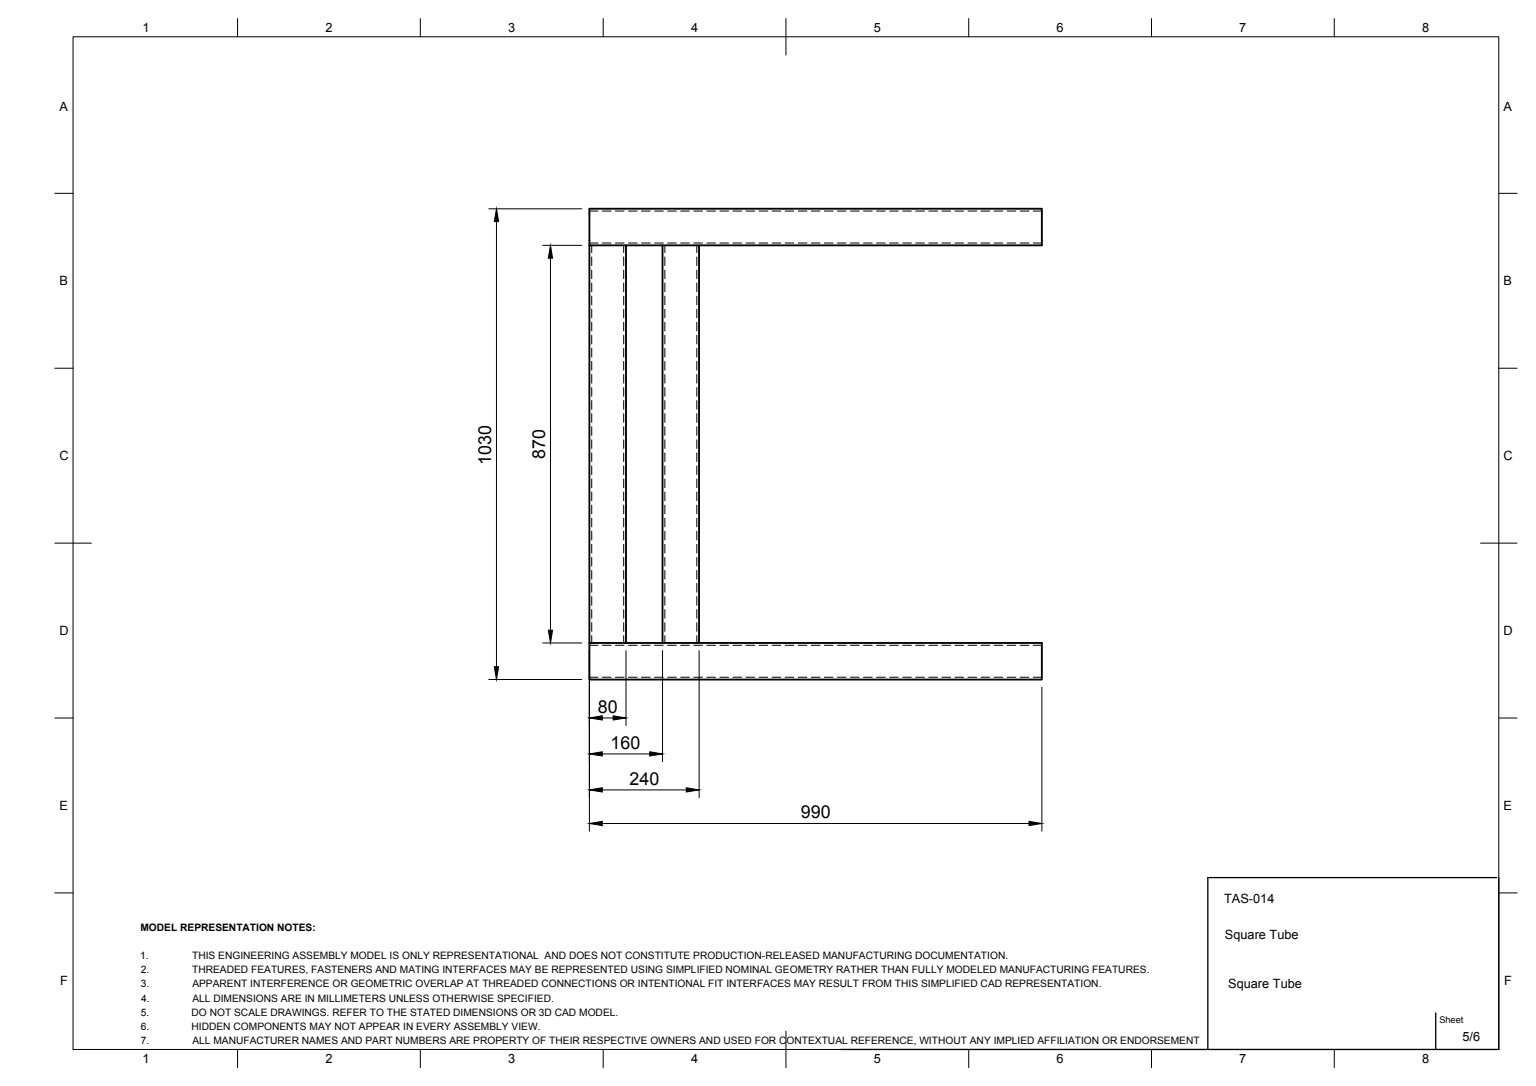
ISO-10303-21;
HEADER;
/* Generated by software containing ST-Developer
 * from STEP Tools, Inc. (www.steptools.com) 
 */

FILE_DESCRIPTION(
/* description */ ('STEP AP214'),
/* implementation_level */ '2;1');

FILE_NAME(
/* name */ 'Square Tube.step',
/* time_stamp */ '2026-11-15T15:22:30-08:00',
/* author */ (''),
/* organization */ (''),
/* preprocessor_version */ 'ST-DEVELOPER v20.2',
/* originating_system */ 'Autodesk Translation Framework v15.17.0.0',
/* authorisation */ '');

FILE_SCHEMA (('AUTOMOTIVE_DESIGN { 1 0 10303 214 3 1 1 }'));
ENDSEC;

DATA;
#10=MECHANICAL_DESIGN_GEOMETRIC_PRESENTATION_REPRESENTATION('',(#79,#80,#81,#82,#83,#84),#3119);
#67=SHAPE_REPRESENTATION_RELATIONSHIP('SRR','None',#3149,#71);
#71=ADVANCED_BREP_SHAPE_REPRESENTATION('',(#88,#89,#90,#91),#3115);
#75=OPEN_SHELL('',(#1779));
#76=OPEN_SHELL('',(#1780));
#77=SHELL_BASED_SURFACE_MODEL('Body5',(#75));
#78=SHELL_BASED_SURFACE_MODEL('Body6',(#76));
#79=STYLED_ITEM('',(#3178),#88);
#80=STYLED_ITEM('',(#3178),#89);
#81=STYLED_ITEM('',(#3178),#90);
#82=STYLED_ITEM('',(#3178),#91);
#83=STYLED_ITEM('',(#3178),#77);
#84=STYLED_ITEM('',(#3178),#78);
#88=MANIFOLD_SOLID_BREP('Body1',#1800);
#89=MANIFOLD_SOLID_BREP('Body2',#1801);
#90=MANIFOLD_SOLID_BREP('Body3',#1802);
#91=MANIFOLD_SOLID_BREP('Body4',#1803);
#95=FACE_BOUND('',#317,.T.);
#96=FACE_BOUND('',#319,.T.);
#97=FACE_BOUND('',#337,.T.);
#98=FACE_BOUND('',#339,.T.);
#99=FACE_BOUND('',#357,.T.);
#100=FACE_BOUND('',#359,.T.);
#101=FACE_BOUND('',#377,.T.);
#102=FACE_BOUND('',#379,.T.);
#103=CIRCLE('',#1856,5.);
#104=CIRCLE('',#1857,5.);
#105=CIRCLE('',#1860,5.);
#106=CIRCLE('',#1861,5.);
#107=CIRCLE('',#1864,5.);
#108=CIRCLE('',#1865,5.);
#109=CIRCLE('',#1868,5.);
#110=CIRCLE('',#1869,5.);
#111=CIRCLE('',#1872,10.);
#112=CIRCLE('',#1873,10.);
#113=CIRCLE('',#1876,10.);
#114=CIRCLE('',#1877,10.);
#115=CIRCLE('',#1880,10.);
#116=CIRCLE('',#1881,10.);
#117=CIRCLE('',#1884,10.);
#118=CIRCLE('',#1885,10.);
#119=CIRCLE('',#1890,5.);
#120=CIRCLE('',#1891,5.);
#121=CIRCLE('',#1894,5.);
#122=CIRCLE('',#1895,5.);
#123=CIRCLE('',#1898,5.);
#124=CIRCLE('',#1899,5.);
#125=CIRCLE('',#1902,5.);
#126=CIRCLE('',#1903,5.);
#127=CIRCLE('',#1906,10.);
#128=CIRCLE('',#1907,10.);
#129=CIRCLE('',#1910,10.);
#130=CIRCLE('',#1911,10.);
#131=CIRCLE('',#1914,10.);
#132=CIRCLE('',#1915,10.);
#133=CIRCLE('',#1918,10.);
#134=CIRCLE('',#1919,10.);
#135=CIRCLE('',#1923,10.);
#136=CIRCLE('',#1924,10.);
#137=CIRCLE('',#1927,10.);
#138=CIRCLE('',#1928,10.);
#139=CIRCLE('',#1931,10.);
#140=CIRCLE('',#1932,10.);
#141=CIRCLE('',#1935,10.);
#142=CIRCLE('',#1936,10.);
#143=CIRCLE('',#1938,5.);
#144=CIRCLE('',#1939,5.);
#145=CIRCLE('',#1942,5.);
#146=CIRCLE('',#1943,5.);
#147=CIRCLE('',#1946,5.);
#148=CIRCLE('',#1947,5.);
#149=CIRCLE('',#1950,5.);
#150=CIRCLE('',#1951,5.);
#151=CIRCLE('',#1957,10.);
#152=CIRCLE('',#1958,10.);
#153=CIRCLE('',#1961,10.);
#154=CIRCLE('',#1962,10.);
#155=CIRCLE('',#1965,10.);
#156=CIRCLE('',#1966,10.);
#157=CIRCLE('',#1969,10.);
#158=CIRCLE('',#1970,10.);
#159=CIRCLE('',#1972,5.);
#160=CIRCLE('',#1973,5.);
#161=CIRCLE('',#1976,5.);
#162=CIRCLE('',#1977,5.);
#163=CIRCLE('',#1980,5.);
#164=CIRCLE('',#1981,5.);
#165=CIRCLE('',#1984,5.);
#166=CIRCLE('',#1985,5.);
#167=CIRCLE('',#1991,5.);
#168=CIRCLE('',#1992,5.);
#169=CIRCLE('',#1993,5.);
#170=CIRCLE('',#1994,5.);
#171=CIRCLE('',#1996,5.);
#172=CIRCLE('',#1997,5.);
#173=CIRCLE('',#1998,5.);
#174=CIRCLE('',#1999,5.);
#175=CYLINDRICAL_SURFACE('',#1855,5.);
#176=CYLINDRICAL_SURFACE('',#1859,5.);
#177=CYLINDRICAL_SURFACE('',#1863,5.);
#178=CYLINDRICAL_SURFACE('',#1867,5.);
#179=CYLINDRICAL_SURFACE('',#1871,10.);
#180=CYLINDRICAL_SURFACE('',#1875,10.);
#181=CYLINDRICAL_SURFACE('',#1879,10.);
#182=CYLINDRICAL_SURFACE('',#1883,10.);
#183=CYLINDRICAL_SURFACE('',#1889,5.);
#184=CYLINDRICAL_SURFACE('',#1893,5.);
#185=CYLINDRICAL_SURFACE('',#1897,5.);
#186=CYLINDRICAL_SURFACE('',#1901,5.);
#187=CYLINDRICAL_SURFACE('',#1905,10.);
#188=CYLINDRICAL_SURFACE('',#1909,10.);
#189=CYLINDRICAL_SURFACE('',#1913,10.);
#190=CYLINDRICAL_SURFACE('',#1917,10.);
#191=CYLINDRICAL_SURFACE('',#1922,10.);
#192=CYLINDRICAL_SURFACE('',#1926,10.);
#193=CYLINDRICAL_SURFACE('',#1930,10.);
#194=CYLINDRICAL_SURFACE('',#1934,10.);
#195=CYLINDRICAL_SURFACE('',#1937,5.);
#196=CYLINDRICAL_SURFACE('',#1941,5.);
#197=CYLINDRICAL_SURFACE('',#1945,5.);
#198=CYLINDRICAL_SURFACE('',#1949,5.);
#199=CYLINDRICAL_SURFACE('',#1956,10.);
#200=CYLINDRICAL_SURFACE('',#1960,10.);
#201=CYLINDRICAL_SURFACE('',#1964,10.);
#202=CYLINDRICAL_SURFACE('',#1968,10.);
#203=CYLINDRICAL_SURFACE('',#1971,5.);
#204=CYLINDRICAL_SURFACE('',#1975,5.);
#205=CYLINDRICAL_SURFACE('',#1979,5.);
#206=CYLINDRICAL_SURFACE('',#1983,5.);
#207=FACE_OUTER_BOUND('',#300,.T.);
#208=FACE_OUTER_BOUND('',#301,.T.);
#209=FACE_OUTER_BOUND('',#302,.T.);
#210=FACE_OUTER_BOUND('',#303,.T.);
#211=FACE_OUTER_BOUND('',#304,.T.);
#212=FACE_OUTER_BOUND('',#305,.T.);
#213=FACE_OUTER_BOUND('',#306,.T.);
#214=FACE_OUTER_BOUND('',#307,.T.);
#215=FACE_OUTER_BOUND('',#308,.T.);
#216=FACE_OUTER_BOUND('',#309,.T.);
#217=FACE_OUTER_BOUND('',#310,.T.);
#218=FACE_OUTER_BOUND('',#311,.T.);
#219=FACE_OUTER_BOUND('',#312,.T.);
#220=FACE_OUTER_BOUND('',#313,.T.);
#221=FACE_OUTER_BOUND('',#314,.T.);
#222=FACE_OUTER_BOUND('',#315,.T.);
#223=FACE_OUTER_BOUND('',#316,.T.);
#224=FACE_OUTER_BOUND('',#318,.T.);
#225=FACE_OUTER_BOUND('',#320,.T.);
#226=FACE_OUTER_BOUND('',#321,.T.);
#227=FACE_OUTER_BOUND('',#322,.T.);
#228=FACE_OUTER_BOUND('',#323,.T.);
#229=FACE_OUTER_BOUND('',#324,.T.);
#230=FACE_OUTER_BOUND('',#325,.T.);
#231=FACE_OUTER_BOUND('',#326,.T.);
#232=FACE_OUTER_BOUND('',#327,.T.);
#233=FACE_OUTER_BOUND('',#328,.T.);
#234=FACE_OUTER_BOUND('',#329,.T.);
#235=FACE_OUTER_BOUND('',#330,.T.);
#236=FACE_OUTER_BOUND('',#331,.T.);
#237=FACE_OUTER_BOUND('',#332,.T.);
#238=FACE_OUTER_BOUND('',#333,.T.);
#239=FACE_OUTER_BOUND('',#334,.T.);
#240=FACE_OUTER_BOUND('',#335,.T.);
#241=FACE_OUTER_BOUND('',#336,.T.);
#242=FACE_OUTER_BOUND('',#338,.T.);
#243=FACE_OUTER_BOUND('',#340,.T.);
#244=FACE_OUTER_BOUND('',#341,.T.);
#245=FACE_OUTER_BOUND('',#342,.T.);
#246=FACE_OUTER_BOUND('',#343,.T.);
#247=FACE_OUTER_BOUND('',#344,.T.);
#248=FACE_OUTER_BOUND('',#345,.T.);
#249=FACE_OUTER_BOUND('',#346,.T.);
#250=FACE_OUTER_BOUND('',#347,.T.);
#251=FACE_OUTER_BOUND('',#348,.T.);
#252=FACE_OUTER_BOUND('',#349,.T.);
#253=FACE_OUTER_BOUND('',#350,.T.);
#254=FACE_OUTER_BOUND('',#351,.T.);
#255=FACE_OUTER_BOUND('',#352,.T.);
#256=FACE_OUTER_BOUND('',#353,.T.);
#257=FACE_OUTER_BOUND('',#354,.T.);
#258=FACE_OUTER_BOUND('',#355,.T.);
#259=FACE_OUTER_BOUND('',#356,.T.);
#260=FACE_OUTER_BOUND('',#358,.T.);
#261=FACE_OUTER_BOUND('',#360,.T.);
#262=FACE_OUTER_BOUND('',#361,.T.);
#263=FACE_OUTER_BOUND('',#362,.T.);
#264=FACE_OUTER_BOUND('',#363,.T.);
#265=FACE_OUTER_BOUND('',#364,.T.);
#266=FACE_OUTER_BOUND('',#365,.T.);
#267=FACE_OUTER_BOUND('',#366,.T.);
#268=FACE_OUTER_BOUND('',#367,.T.);
#269=FACE_OUTER_BOUND('',#368,.T.);
#270=FACE_OUTER_BOUND('',#369,.T.);
#271=FACE_OUTER_BOUND('',#370,.T.);
#272=FACE_OUTER_BOUND('',#371,.T.);
#273=FACE_OUTER_BOUND('',#372,.T.);
#274=FACE_OUTER_BOUND('',#373,.T.);
#275=FACE_OUTER_BOUND('',#374,.T.);
#276=FACE_OUTER_BOUND('',#375,.T.);
#277=FACE_OUTER_BOUND('',#376,.T.);
#278=FACE_OUTER_BOUND('',#378,.T.);
#279=FACE_OUTER_BOUND('',#380,.T.);
#280=FACE_OUTER_BOUND('',#381,.T.);
#300=EDGE_LOOP('',(#1168,#1169,#1170,#1171));
#301=EDGE_LOOP('',(#1172,#1173,#1174,#1175));
#302=EDGE_LOOP('',(#1176,#1177,#1178,#1179));
#303=EDGE_LOOP('',(#1180,#1181,#1182,#1183));
#304=EDGE_LOOP('',(#1184,#1185,#1186,#1187));
#305=EDGE_LOOP('',(#1188,#1189,#1190,#1191));
#306=EDGE_LOOP('',(#1192,#1193,#1194,#1195));
#307=EDGE_LOOP('',(#1196,#1197,#1198,#1199));
#308=EDGE_LOOP('',(#1200,#1201,#1202,#1203));
#309=EDGE_LOOP('',(#1204,#1205,#1206,#1207));
#310=EDGE_LOOP('',(#1208,#1209,#1210,#1211));
#311=EDGE_LOOP('',(#1212,#1213,#1214,#1215));
#312=EDGE_LOOP('',(#1216,#1217,#1218,#1219));
#313=EDGE_LOOP('',(#1220,#1221,#1222,#1223));
#314=EDGE_LOOP('',(#1224,#1225,#1226,#1227));
#315=EDGE_LOOP('',(#1228,#1229,#1230,#1231));
#316=EDGE_LOOP('',(#1232,#1233,#1234,#1235,#1236,#1237,#1238,#1239));
#317=EDGE_LOOP('',(#1240,#1241,#1242,#1243,#1244,#1245,#1246,#1247));
#318=EDGE_LOOP('',(#1248,#1249,#1250,#1251,#1252,#1253,#1254,#1255));
#319=EDGE_LOOP('',(#1256,#1257,#1258,#1259,#1260,#1261,#1262,#1263));
#320=EDGE_LOOP('',(#1264,#1265,#1266,#1267));
#321=EDGE_LOOP('',(#1268,#1269,#1270,#1271));
#322=EDGE_LOOP('',(#1272,#1273,#1274,#1275));
#323=EDGE_LOOP('',(#1276,#1277,#1278,#1279));
#324=EDGE_LOOP('',(#1280,#1281,#1282,#1283));
#325=EDGE_LOOP('',(#1284,#1285,#1286,#1287));
#326=EDGE_LOOP('',(#1288,#1289,#1290,#1291));
#327=EDGE_LOOP('',(#1292,#1293,#1294,#1295));
#328=EDGE_LOOP('',(#1296,#1297,#1298,#1299));
#329=EDGE_LOOP('',(#1300,#1301,#1302,#1303));
#330=EDGE_LOOP('',(#1304,#1305,#1306,#1307));
#331=EDGE_LOOP('',(#1308,#1309,#1310,#1311));
#332=EDGE_LOOP('',(#1312,#1313,#1314,#1315));
#333=EDGE_LOOP('',(#1316,#1317,#1318,#1319));
#334=EDGE_LOOP('',(#1320,#1321,#1322,#1323));
#335=EDGE_LOOP('',(#1324,#1325,#1326,#1327));
#336=EDGE_LOOP('',(#1328,#1329,#1330,#1331,#1332,#1333,#1334,#1335));
#337=EDGE_LOOP('',(#1336,#1337,#1338,#1339,#1340,#1341,#1342,#1343));
#338=EDGE_LOOP('',(#1344,#1345,#1346,#1347,#1348,#1349,#1350,#1351));
#339=EDGE_LOOP('',(#1352,#1353,#1354,#1355,#1356,#1357,#1358,#1359));
#340=EDGE_LOOP('',(#1360,#1361,#1362,#1363));
#341=EDGE_LOOP('',(#1364,#1365,#1366,#1367));
#342=EDGE_LOOP('',(#1368,#1369,#1370,#1371));
#343=EDGE_LOOP('',(#1372,#1373,#1374,#1375));
#344=EDGE_LOOP('',(#1376,#1377,#1378,#1379));
#345=EDGE_LOOP('',(#1380,#1381,#1382,#1383));
#346=EDGE_LOOP('',(#1384,#1385,#1386,#1387));
#347=EDGE_LOOP('',(#1388,#1389,#1390,#1391));
#348=EDGE_LOOP('',(#1392,#1393,#1394,#1395));
#349=EDGE_LOOP('',(#1396,#1397,#1398,#1399));
#350=EDGE_LOOP('',(#1400,#1401,#1402,#1403));
#351=EDGE_LOOP('',(#1404,#1405,#1406,#1407));
#352=EDGE_LOOP('',(#1408,#1409,#1410,#1411));
#353=EDGE_LOOP('',(#1412,#1413,#1414,#1415));
#354=EDGE_LOOP('',(#1416,#1417,#1418,#1419));
#355=EDGE_LOOP('',(#1420,#1421,#1422,#1423));
#356=EDGE_LOOP('',(#1424,#1425,#1426,#1427,#1428,#1429,#1430,#1431));
#357=EDGE_LOOP('',(#1432,#1433,#1434,#1435,#1436,#1437,#1438,#1439));
#358=EDGE_LOOP('',(#1440,#1441,#1442,#1443,#1444,#1445,#1446,#1447));
#359=EDGE_LOOP('',(#1448,#1449,#1450,#1451,#1452,#1453,#1454,#1455));
#360=EDGE_LOOP('',(#1456,#1457,#1458,#1459));
#361=EDGE_LOOP('',(#1460,#1461,#1462,#1463));
#362=EDGE_LOOP('',(#1464,#1465,#1466,#1467));
#363=EDGE_LOOP('',(#1468,#1469,#1470,#1471));
#364=EDGE_LOOP('',(#1472,#1473,#1474,#1475));
#365=EDGE_LOOP('',(#1476,#1477,#1478,#1479));
#366=EDGE_LOOP('',(#1480,#1481,#1482,#1483));
#367=EDGE_LOOP('',(#1484,#1485,#1486,#1487));
#368=EDGE_LOOP('',(#1488,#1489,#1490,#1491));
#369=EDGE_LOOP('',(#1492,#1493,#1494,#1495));
#370=EDGE_LOOP('',(#1496,#1497,#1498,#1499));
#371=EDGE_LOOP('',(#1500,#1501,#1502,#1503));
#372=EDGE_LOOP('',(#1504,#1505,#1506,#1507));
#373=EDGE_LOOP('',(#1508,#1509,#1510,#1511));
#374=EDGE_LOOP('',(#1512,#1513,#1514,#1515));
#375=EDGE_LOOP('',(#1516,#1517,#1518,#1519));
#376=EDGE_LOOP('',(#1520,#1521,#1522,#1523,#1524,#1525,#1526,#1527));
#377=EDGE_LOOP('',(#1528,#1529,#1530,#1531,#1532,#1533,#1534,#1535));
#378=EDGE_LOOP('',(#1536,#1537,#1538,#1539,#1540,#1541,#1542,#1543));
#379=EDGE_LOOP('',(#1544,#1545,#1546,#1547,#1548,#1549,#1550,#1551));
#380=EDGE_LOOP('',(#1552,#1553,#1554,#1555,#1556,#1557,#1558,#1559));
#381=EDGE_LOOP('',(#1560,#1561,#1562,#1563,#1564,#1565,#1566,#1567));
#401=LINE('',#2584,#576);
#402=LINE('',#2586,#577);
#403=LINE('',#2588,#578);
#404=LINE('',#2589,#579);
#405=LINE('',#2593,#580);
#406=LINE('',#2599,#581);
#407=LINE('',#2600,#582);
#408=LINE('',#2601,#583);
#409=LINE('',#2605,#584);
#410=LINE('',#2611,#585);
#411=LINE('',#2612,#586);
#412=LINE('',#2613,#587);
#413=LINE('',#2617,#588);
#414=LINE('',#2623,#589);
#415=LINE('',#2624,#590);
#416=LINE('',#2625,#591);
#417=LINE('',#2632,#592);
#418=LINE('',#2634,#593);
#419=LINE('',#2636,#594);
#420=LINE('',#2637,#595);
#421=LINE('',#2643,#596);
#422=LINE('',#2646,#597);
#423=LINE('',#2648,#598);
#424=LINE('',#2649,#599);
#425=LINE('',#2655,#600);
#426=LINE('',#2658,#601);
#427=LINE('',#2660,#602);
#428=LINE('',#2661,#603);
#429=LINE('',#2667,#604);
#430=LINE('',#2670,#605);
#431=LINE('',#2672,#606);
#432=LINE('',#2673,#607);
#433=LINE('',#2682,#608);
#434=LINE('',#2684,#609);
#435=LINE('',#2686,#610);
#436=LINE('',#2687,#611);
#437=LINE('',#2691,#612);
#438=LINE('',#2697,#613);
#439=LINE('',#2698,#614);
#440=LINE('',#2699,#615);
#441=LINE('',#2703,#616);
#442=LINE('',#2709,#617);
#443=LINE('',#2710,#618);
#444=LINE('',#2711,#619);
#445=LINE('',#2715,#620);
#446=LINE('',#2721,#621);
#447=LINE('',#2722,#622);
#448=LINE('',#2723,#623);
#449=LINE('',#2730,#624);
#450=LINE('',#2732,#625);
#451=LINE('',#2734,#626);
#452=LINE('',#2735,#627);
#453=LINE('',#2741,#628);
#454=LINE('',#2744,#629);
#455=LINE('',#2746,#630);
#456=LINE('',#2747,#631);
#457=LINE('',#2753,#632);
#458=LINE('',#2756,#633);
#459=LINE('',#2758,#634);
#460=LINE('',#2759,#635);
#461=LINE('',#2765,#636);
#462=LINE('',#2768,#637);
#463=LINE('',#2770,#638);
#464=LINE('',#2771,#639);
#465=LINE('',#2782,#640);
#466=LINE('',#2785,#641);
#467=LINE('',#2788,#642);
#468=LINE('',#2790,#643);
#469=LINE('',#2791,#644);
#470=LINE('',#2797,#645);
#471=LINE('',#2800,#646);
#472=LINE('',#2802,#647);
#473=LINE('',#2803,#648);
#474=LINE('',#2809,#649);
#475=LINE('',#2812,#650);
#476=LINE('',#2814,#651);
#477=LINE('',#2815,#652);
#478=LINE('',#2821,#653);
#479=LINE('',#2825,#654);
#480=LINE('',#2829,#655);
#481=LINE('',#2834,#656);
#482=LINE('',#2835,#657);
#483=LINE('',#2836,#658);
#484=LINE('',#2840,#659);
#485=LINE('',#2846,#660);
#486=LINE('',#2847,#661);
#487=LINE('',#2848,#662);
#488=LINE('',#2852,#663);
#489=LINE('',#2858,#664);
#490=LINE('',#2859,#665);
#491=LINE('',#2860,#666);
#492=LINE('',#2864,#667);
#493=LINE('',#2868,#668);
#494=LINE('',#2869,#669);
#495=LINE('',#2871,#670);
#496=LINE('',#2872,#671);
#497=LINE('',#2880,#672);
#498=LINE('',#2883,#673);
#499=LINE('',#2886,#674);
#500=LINE('',#2888,#675);
#501=LINE('',#2889,#676);
#502=LINE('',#2895,#677);
#503=LINE('',#2898,#678);
#504=LINE('',#2900,#679);
#505=LINE('',#2901,#680);
#506=LINE('',#2907,#681);
#507=LINE('',#2910,#682);
#508=LINE('',#2912,#683);
#509=LINE('',#2913,#684);
#510=LINE('',#2919,#685);
#511=LINE('',#2923,#686);
#512=LINE('',#2927,#687);
#513=LINE('',#2932,#688);
#514=LINE('',#2933,#689);
#515=LINE('',#2934,#690);
#516=LINE('',#2938,#691);
#517=LINE('',#2944,#692);
#518=LINE('',#2945,#693);
#519=LINE('',#2946,#694);
#520=LINE('',#2950,#695);
#521=LINE('',#2956,#696);
#522=LINE('',#2957,#697);
#523=LINE('',#2958,#698);
#524=LINE('',#2962,#699);
#525=LINE('',#2966,#700);
#526=LINE('',#2967,#701);
#527=LINE('',#2969,#702);
#528=LINE('',#2970,#703);
#529=LINE('',#2978,#704);
#530=LINE('',#2982,#705);
#531=LINE('',#2986,#706);
#532=LINE('',#2989,#707);
#533=LINE('',#2993,#708);
#534=LINE('',#2997,#709);
#535=LINE('',#3001,#710);
#536=LINE('',#3005,#711);
#576=VECTOR('',#2042,1000.);
#577=VECTOR('',#2043,1000.);
#578=VECTOR('',#2044,1000.);
#579=VECTOR('',#2045,1000.);
#580=VECTOR('',#2048,1000.);
#581=VECTOR('',#2055,1000.);
#582=VECTOR('',#2056,1000.);
#583=VECTOR('',#2057,1000.);
#584=VECTOR('',#2060,1000.);
#585=VECTOR('',#2067,1000.);
#586=VECTOR('',#2068,1000.);
#587=VECTOR('',#2069,1000.);
#588=VECTOR('',#2072,1000.);
#589=VECTOR('',#2079,1000.);
#590=VECTOR('',#2080,1000.);
#591=VECTOR('',#2081,1000.);
#592=VECTOR('',#2090,1000.);
#593=VECTOR('',#2091,1000.);
#594=VECTOR('',#2092,1000.);
#595=VECTOR('',#2093,1000.);
#596=VECTOR('',#2100,1000.);
#597=VECTOR('',#2103,1000.);
#598=VECTOR('',#2104,1000.);
#599=VECTOR('',#2105,1000.);
#600=VECTOR('',#2112,1000.);
#601=VECTOR('',#2115,1000.);
#602=VECTOR('',#2116,1000.);
#603=VECTOR('',#2117,1000.);
#604=VECTOR('',#2124,1000.);
#605=VECTOR('',#2127,1000.);
#606=VECTOR('',#2128,1000.);
#607=VECTOR('',#2129,1000.);
#608=VECTOR('',#2142,1000.);
#609=VECTOR('',#2143,1000.);
#610=VECTOR('',#2144,1000.);
#611=VECTOR('',#2145,1000.);
#612=VECTOR('',#2148,1000.);
#613=VECTOR('',#2155,1000.);
#614=VECTOR('',#2156,1000.);
#615=VECTOR('',#2157,1000.);
#616=VECTOR('',#2160,1000.);
#617=VECTOR('',#2167,1000.);
#618=VECTOR('',#2168,1000.);
#619=VECTOR('',#2169,1000.);
#620=VECTOR('',#2172,1000.);
#621=VECTOR('',#2179,1000.);
#622=VECTOR('',#2180,1000.);
#623=VECTOR('',#2181,1000.);
#624=VECTOR('',#2190,1000.);
#625=VECTOR('',#2191,1000.);
#626=VECTOR('',#2192,1000.);
#627=VECTOR('',#2193,1000.);
#628=VECTOR('',#2200,1000.);
#629=VECTOR('',#2203,1000.);
#630=VECTOR('',#2204,1000.);
#631=VECTOR('',#2205,1000.);
#632=VECTOR('',#2212,1000.);
#633=VECTOR('',#2215,1000.);
#634=VECTOR('',#2216,1000.);
#635=VECTOR('',#2217,1000.);
#636=VECTOR('',#2224,1000.);
#637=VECTOR('',#2227,1000.);
#638=VECTOR('',#2228,1000.);
#639=VECTOR('',#2229,1000.);
#640=VECTOR('',#2244,1000.);
#641=VECTOR('',#2247,1000.);
#642=VECTOR('',#2250,1000.);
#643=VECTOR('',#2251,1000.);
#644=VECTOR('',#2252,1000.);
#645=VECTOR('',#2259,1000.);
#646=VECTOR('',#2262,1000.);
#647=VECTOR('',#2263,1000.);
#648=VECTOR('',#2264,1000.);
#649=VECTOR('',#2271,1000.);
#650=VECTOR('',#2274,1000.);
#651=VECTOR('',#2275,1000.);
#652=VECTOR('',#2276,1000.);
#653=VECTOR('',#2283,1000.);
#654=VECTOR('',#2286,1000.);
#655=VECTOR('',#2289,1000.);
#656=VECTOR('',#2294,1000.);
#657=VECTOR('',#2295,1000.);
#658=VECTOR('',#2296,1000.);
#659=VECTOR('',#2299,1000.);
#660=VECTOR('',#2306,1000.);
#661=VECTOR('',#2307,1000.);
#662=VECTOR('',#2308,1000.);
#663=VECTOR('',#2311,1000.);
#664=VECTOR('',#2318,1000.);
#665=VECTOR('',#2319,1000.);
#666=VECTOR('',#2320,1000.);
#667=VECTOR('',#2323,1000.);
#668=VECTOR('',#2330,1000.);
#669=VECTOR('',#2331,1000.);
#670=VECTOR('',#2334,1000.);
#671=VECTOR('',#2335,1000.);
#672=VECTOR('',#2344,1000.);
#673=VECTOR('',#2347,1000.);
#674=VECTOR('',#2350,1000.);
#675=VECTOR('',#2351,1000.);
#676=VECTOR('',#2352,1000.);
#677=VECTOR('',#2359,1000.);
#678=VECTOR('',#2362,1000.);
#679=VECTOR('',#2363,1000.);
#680=VECTOR('',#2364,1000.);
#681=VECTOR('',#2371,1000.);
#682=VECTOR('',#2374,1000.);
#683=VECTOR('',#2375,1000.);
#684=VECTOR('',#2376,1000.);
#685=VECTOR('',#2383,1000.);
#686=VECTOR('',#2386,1000.);
#687=VECTOR('',#2389,1000.);
#688=VECTOR('',#2394,1000.);
#689=VECTOR('',#2395,1000.);
#690=VECTOR('',#2396,1000.);
#691=VECTOR('',#2399,1000.);
#692=VECTOR('',#2406,1000.);
#693=VECTOR('',#2407,1000.);
#694=VECTOR('',#2408,1000.);
#695=VECTOR('',#2411,1000.);
#696=VECTOR('',#2418,1000.);
#697=VECTOR('',#2419,1000.);
#698=VECTOR('',#2420,1000.);
#699=VECTOR('',#2423,1000.);
#700=VECTOR('',#2430,1000.);
#701=VECTOR('',#2431,1000.);
#702=VECTOR('',#2434,1000.);
#703=VECTOR('',#2435,1000.);
#704=VECTOR('',#2444,1000.);
#705=VECTOR('',#2447,1000.);
#706=VECTOR('',#2450,1000.);
#707=VECTOR('',#2453,1000.);
#708=VECTOR('',#2456,1000.);
#709=VECTOR('',#2459,1000.);
#710=VECTOR('',#2462,1000.);
#711=VECTOR('',#2465,1000.);
#751=VERTEX_POINT('',#2582);
#752=VERTEX_POINT('',#2583);
#753=VERTEX_POINT('',#2585);
#754=VERTEX_POINT('',#2587);
#755=VERTEX_POINT('',#2591);
#756=VERTEX_POINT('',#2592);
#757=VERTEX_POINT('',#2597);
#758=VERTEX_POINT('',#2598);
#759=VERTEX_POINT('',#2603);
#760=VERTEX_POINT('',#2604);
#761=VERTEX_POINT('',#2609);
#762=VERTEX_POINT('',#2610);
#763=VERTEX_POINT('',#2615);
#764=VERTEX_POINT('',#2616);
#765=VERTEX_POINT('',#2621);
#766=VERTEX_POINT('',#2622);
#767=VERTEX_POINT('',#2630);
#768=VERTEX_POINT('',#2631);
#769=VERTEX_POINT('',#2633);
#770=VERTEX_POINT('',#2635);
#771=VERTEX_POINT('',#2639);
#772=VERTEX_POINT('',#2641);
#773=VERTEX_POINT('',#2645);
#774=VERTEX_POINT('',#2647);
#775=VERTEX_POINT('',#2651);
#776=VERTEX_POINT('',#2653);
#777=VERTEX_POINT('',#2657);
#778=VERTEX_POINT('',#2659);
#779=VERTEX_POINT('',#2663);
#780=VERTEX_POINT('',#2665);
#781=VERTEX_POINT('',#2669);
#782=VERTEX_POINT('',#2671);
#783=VERTEX_POINT('',#2680);
#784=VERTEX_POINT('',#2681);
#785=VERTEX_POINT('',#2683);
#786=VERTEX_POINT('',#2685);
#787=VERTEX_POINT('',#2689);
#788=VERTEX_POINT('',#2690);
#789=VERTEX_POINT('',#2695);
#790=VERTEX_POINT('',#2696);
#791=VERTEX_POINT('',#2701);
#792=VERTEX_POINT('',#2702);
#793=VERTEX_POINT('',#2707);
#794=VERTEX_POINT('',#2708);
#795=VERTEX_POINT('',#2713);
#796=VERTEX_POINT('',#2714);
#797=VERTEX_POINT('',#2719);
#798=VERTEX_POINT('',#2720);
#799=VERTEX_POINT('',#2728);
#800=VERTEX_POINT('',#2729);
#801=VERTEX_POINT('',#2731);
#802=VERTEX_POINT('',#2733);
#803=VERTEX_POINT('',#2737);
#804=VERTEX_POINT('',#2739);
#805=VERTEX_POINT('',#2743);
#806=VERTEX_POINT('',#2745);
#807=VERTEX_POINT('',#2749);
#808=VERTEX_POINT('',#2751);
#809=VERTEX_POINT('',#2755);
#810=VERTEX_POINT('',#2757);
#811=VERTEX_POINT('',#2761);
#812=VERTEX_POINT('',#2763);
#813=VERTEX_POINT('',#2767);
#814=VERTEX_POINT('',#2769);
#815=VERTEX_POINT('',#2778);
#816=VERTEX_POINT('',#2779);
#817=VERTEX_POINT('',#2781);
#818=VERTEX_POINT('',#2783);
#819=VERTEX_POINT('',#2787);
#820=VERTEX_POINT('',#2789);
#821=VERTEX_POINT('',#2793);
#822=VERTEX_POINT('',#2795);
#823=VERTEX_POINT('',#2799);
#824=VERTEX_POINT('',#2801);
#825=VERTEX_POINT('',#2805);
#826=VERTEX_POINT('',#2807);
#827=VERTEX_POINT('',#2811);
#828=VERTEX_POINT('',#2813);
#829=VERTEX_POINT('',#2817);
#830=VERTEX_POINT('',#2819);
#831=VERTEX_POINT('',#2823);
#832=VERTEX_POINT('',#2824);
#833=VERTEX_POINT('',#2826);
#834=VERTEX_POINT('',#2828);
#835=VERTEX_POINT('',#2832);
#836=VERTEX_POINT('',#2833);
#837=VERTEX_POINT('',#2838);
#838=VERTEX_POINT('',#2839);
#839=VERTEX_POINT('',#2844);
#840=VERTEX_POINT('',#2845);
#841=VERTEX_POINT('',#2850);
#842=VERTEX_POINT('',#2851);
#843=VERTEX_POINT('',#2856);
#844=VERTEX_POINT('',#2857);
#845=VERTEX_POINT('',#2862);
#846=VERTEX_POINT('',#2863);
#847=VERTEX_POINT('',#2876);
#848=VERTEX_POINT('',#2877);
#849=VERTEX_POINT('',#2879);
#850=VERTEX_POINT('',#2881);
#851=VERTEX_POINT('',#2885);
#852=VERTEX_POINT('',#2887);
#853=VERTEX_POINT('',#2891);
#854=VERTEX_POINT('',#2893);
#855=VERTEX_POINT('',#2897);
#856=VERTEX_POINT('',#2899);
#857=VERTEX_POINT('',#2903);
#858=VERTEX_POINT('',#2905);
#859=VERTEX_POINT('',#2909);
#860=VERTEX_POINT('',#2911);
#861=VERTEX_POINT('',#2915);
#862=VERTEX_POINT('',#2917);
#863=VERTEX_POINT('',#2921);
#864=VERTEX_POINT('',#2922);
#865=VERTEX_POINT('',#2924);
#866=VERTEX_POINT('',#2926);
#867=VERTEX_POINT('',#2930);
#868=VERTEX_POINT('',#2931);
#869=VERTEX_POINT('',#2936);
#870=VERTEX_POINT('',#2937);
#871=VERTEX_POINT('',#2942);
#872=VERTEX_POINT('',#2943);
#873=VERTEX_POINT('',#2948);
#874=VERTEX_POINT('',#2949);
#875=VERTEX_POINT('',#2954);
#876=VERTEX_POINT('',#2955);
#877=VERTEX_POINT('',#2960);
#878=VERTEX_POINT('',#2961);
#879=VERTEX_POINT('',#2974);
#880=VERTEX_POINT('',#2975);
#881=VERTEX_POINT('',#2977);
#882=VERTEX_POINT('',#2979);
#883=VERTEX_POINT('',#2981);
#884=VERTEX_POINT('',#2983);
#885=VERTEX_POINT('',#2985);
#886=VERTEX_POINT('',#2987);
#887=VERTEX_POINT('',#2991);
#888=VERTEX_POINT('',#2992);
#889=VERTEX_POINT('',#2994);
#890=VERTEX_POINT('',#2996);
#891=VERTEX_POINT('',#2998);
#892=VERTEX_POINT('',#3000);
#893=VERTEX_POINT('',#3002);
#894=VERTEX_POINT('',#3004);
#921=EDGE_CURVE('',#751,#752,#401,.T.);
#922=EDGE_CURVE('',#752,#753,#402,.T.);
#923=EDGE_CURVE('',#754,#753,#403,.T.);
#924=EDGE_CURVE('',#754,#751,#404,.T.);
#925=EDGE_CURVE('',#755,#756,#405,.T.);
#926=EDGE_CURVE('',#756,#752,#103,.T.);
#927=EDGE_CURVE('',#751,#755,#104,.T.);
#928=EDGE_CURVE('',#757,#758,#406,.T.);
#929=EDGE_CURVE('',#758,#756,#407,.T.);
#930=EDGE_CURVE('',#755,#757,#408,.T.);
#931=EDGE_CURVE('',#759,#760,#409,.T.);
#932=EDGE_CURVE('',#760,#758,#105,.T.);
#933=EDGE_CURVE('',#757,#759,#106,.T.);
#934=EDGE_CURVE('',#761,#762,#410,.T.);
#935=EDGE_CURVE('',#762,#760,#411,.T.);
#936=EDGE_CURVE('',#759,#761,#412,.T.);
#937=EDGE_CURVE('',#763,#764,#413,.T.);
#938=EDGE_CURVE('',#764,#762,#107,.T.);
#939=EDGE_CURVE('',#761,#763,#108,.T.);
#940=EDGE_CURVE('',#765,#766,#414,.T.);
#941=EDGE_CURVE('',#766,#764,#415,.T.);
#942=EDGE_CURVE('',#763,#765,#416,.T.);
#943=EDGE_CURVE('',#753,#766,#109,.T.);
#944=EDGE_CURVE('',#765,#754,#110,.T.);
#945=EDGE_CURVE('',#767,#768,#417,.T.);
#946=EDGE_CURVE('',#769,#767,#418,.T.);
#947=EDGE_CURVE('',#770,#769,#419,.T.);
#948=EDGE_CURVE('',#770,#768,#420,.T.);
#949=EDGE_CURVE('',#768,#771,#111,.T.);
#950=EDGE_CURVE('',#772,#770,#112,.T.);
#951=EDGE_CURVE('',#772,#771,#421,.T.);
#952=EDGE_CURVE('',#771,#773,#422,.T.);
#953=EDGE_CURVE('',#772,#774,#423,.T.);
#954=EDGE_CURVE('',#774,#773,#424,.T.);
#955=EDGE_CURVE('',#773,#775,#113,.T.);
#956=EDGE_CURVE('',#776,#774,#114,.T.);
#957=EDGE_CURVE('',#776,#775,#425,.T.);
#958=EDGE_CURVE('',#775,#777,#426,.T.);
#959=EDGE_CURVE('',#778,#776,#427,.T.);
#960=EDGE_CURVE('',#778,#777,#428,.T.);
#961=EDGE_CURVE('',#777,#779,#115,.T.);
#962=EDGE_CURVE('',#780,#778,#116,.T.);
#963=EDGE_CURVE('',#780,#779,#429,.T.);
#964=EDGE_CURVE('',#781,#779,#430,.T.);
#965=EDGE_CURVE('',#782,#780,#431,.T.);
#966=EDGE_CURVE('',#782,#781,#432,.T.);
#967=EDGE_CURVE('',#781,#767,#117,.T.);
#968=EDGE_CURVE('',#769,#782,#118,.T.);
#969=EDGE_CURVE('',#783,#784,#433,.T.);
#970=EDGE_CURVE('',#784,#785,#434,.T.);
#971=EDGE_CURVE('',#786,#785,#435,.T.);
#972=EDGE_CURVE('',#786,#783,#436,.T.);
#973=EDGE_CURVE('',#787,#788,#437,.T.);
#974=EDGE_CURVE('',#788,#784,#119,.T.);
#975=EDGE_CURVE('',#783,#787,#120,.T.);
#976=EDGE_CURVE('',#789,#790,#438,.T.);
#977=EDGE_CURVE('',#790,#788,#439,.T.);
#978=EDGE_CURVE('',#787,#789,#440,.T.);
#979=EDGE_CURVE('',#791,#792,#441,.T.);
#980=EDGE_CURVE('',#792,#790,#121,.T.);
#981=EDGE_CURVE('',#789,#791,#122,.T.);
#982=EDGE_CURVE('',#793,#794,#442,.T.);
#983=EDGE_CURVE('',#794,#792,#443,.T.);
#984=EDGE_CURVE('',#791,#793,#444,.T.);
#985=EDGE_CURVE('',#795,#796,#445,.T.);
#986=EDGE_CURVE('',#796,#794,#123,.T.);
#987=EDGE_CURVE('',#793,#795,#124,.T.);
#988=EDGE_CURVE('',#797,#798,#446,.T.);
#989=EDGE_CURVE('',#798,#796,#447,.T.);
#990=EDGE_CURVE('',#795,#797,#448,.T.);
#991=EDGE_CURVE('',#785,#798,#125,.T.);
#992=EDGE_CURVE('',#797,#786,#126,.T.);
#993=EDGE_CURVE('',#799,#800,#449,.T.);
#994=EDGE_CURVE('',#801,#799,#450,.T.);
#995=EDGE_CURVE('',#802,#801,#451,.T.);
#996=EDGE_CURVE('',#802,#800,#452,.T.);
#997=EDGE_CURVE('',#800,#803,#127,.T.);
#998=EDGE_CURVE('',#804,#802,#128,.T.);
#999=EDGE_CURVE('',#804,#803,#453,.T.);
#1000=EDGE_CURVE('',#803,#805,#454,.T.);
#1001=EDGE_CURVE('',#804,#806,#455,.T.);
#1002=EDGE_CURVE('',#806,#805,#456,.T.);
#1003=EDGE_CURVE('',#805,#807,#129,.T.);
#1004=EDGE_CURVE('',#808,#806,#130,.T.);
#1005=EDGE_CURVE('',#808,#807,#457,.T.);
#1006=EDGE_CURVE('',#807,#809,#458,.T.);
#1007=EDGE_CURVE('',#810,#808,#459,.T.);
#1008=EDGE_CURVE('',#810,#809,#460,.T.);
#1009=EDGE_CURVE('',#809,#811,#131,.T.);
#1010=EDGE_CURVE('',#812,#810,#132,.T.);
#1011=EDGE_CURVE('',#812,#811,#461,.T.);
#1012=EDGE_CURVE('',#813,#811,#462,.T.);
#1013=EDGE_CURVE('',#814,#812,#463,.T.);
#1014=EDGE_CURVE('',#814,#813,#464,.T.);
#1015=EDGE_CURVE('',#813,#799,#133,.T.);
#1016=EDGE_CURVE('',#801,#814,#134,.T.);
#1017=EDGE_CURVE('',#815,#816,#135,.T.);
#1018=EDGE_CURVE('',#815,#817,#465,.T.);
#1019=EDGE_CURVE('',#817,#818,#136,.T.);
#1020=EDGE_CURVE('',#816,#818,#466,.T.);
#1021=EDGE_CURVE('',#816,#819,#467,.T.);
#1022=EDGE_CURVE('',#818,#820,#468,.T.);
#1023=EDGE_CURVE('',#819,#820,#469,.T.);
#1024=EDGE_CURVE('',#819,#821,#137,.T.);
#1025=EDGE_CURVE('',#820,#822,#138,.T.);
#1026=EDGE_CURVE('',#821,#822,#470,.T.);
#1027=EDGE_CURVE('',#821,#823,#471,.T.);
#1028=EDGE_CURVE('',#822,#824,#472,.T.);
#1029=EDGE_CURVE('',#823,#824,#473,.T.);
#1030=EDGE_CURVE('',#823,#825,#139,.T.);
#1031=EDGE_CURVE('',#824,#826,#140,.T.);
#1032=EDGE_CURVE('',#825,#826,#474,.T.);
#1033=EDGE_CURVE('',#825,#827,#475,.T.);
#1034=EDGE_CURVE('',#826,#828,#476,.T.);
#1035=EDGE_CURVE('',#827,#828,#477,.T.);
#1036=EDGE_CURVE('',#827,#829,#141,.T.);
#1037=EDGE_CURVE('',#828,#830,#142,.T.);
#1038=EDGE_CURVE('',#829,#830,#478,.T.);
#1039=EDGE_CURVE('',#831,#832,#479,.T.);
#1040=EDGE_CURVE('',#831,#833,#143,.T.);
#1041=EDGE_CURVE('',#833,#834,#480,.T.);
#1042=EDGE_CURVE('',#832,#834,#144,.T.);
#1043=EDGE_CURVE('',#835,#836,#481,.T.);
#1044=EDGE_CURVE('',#835,#831,#482,.T.);
#1045=EDGE_CURVE('',#836,#832,#483,.T.);
#1046=EDGE_CURVE('',#837,#838,#484,.T.);
#1047=EDGE_CURVE('',#837,#835,#145,.T.);
#1048=EDGE_CURVE('',#838,#836,#146,.T.);
#1049=EDGE_CURVE('',#839,#840,#485,.T.);
#1050=EDGE_CURVE('',#839,#837,#486,.T.);
#1051=EDGE_CURVE('',#840,#838,#487,.T.);
#1052=EDGE_CURVE('',#841,#842,#488,.T.);
#1053=EDGE_CURVE('',#841,#839,#147,.T.);
#1054=EDGE_CURVE('',#842,#840,#148,.T.);
#1055=EDGE_CURVE('',#843,#844,#489,.T.);
#1056=EDGE_CURVE('',#843,#841,#490,.T.);
#1057=EDGE_CURVE('',#844,#842,#491,.T.);
#1058=EDGE_CURVE('',#845,#846,#492,.T.);
#1059=EDGE_CURVE('',#845,#843,#149,.T.);
#1060=EDGE_CURVE('',#846,#844,#150,.T.);
#1061=EDGE_CURVE('',#833,#845,#493,.T.);
#1062=EDGE_CURVE('',#834,#846,#494,.T.);
#1063=EDGE_CURVE('',#829,#815,#495,.T.);
#1064=EDGE_CURVE('',#830,#817,#496,.T.);
#1065=EDGE_CURVE('',#847,#848,#151,.T.);
#1066=EDGE_CURVE('',#847,#849,#497,.T.);
#1067=EDGE_CURVE('',#849,#850,#152,.T.);
#1068=EDGE_CURVE('',#848,#850,#498,.T.);
#1069=EDGE_CURVE('',#848,#851,#499,.T.);
#1070=EDGE_CURVE('',#850,#852,#500,.T.);
#1071=EDGE_CURVE('',#851,#852,#501,.T.);
#1072=EDGE_CURVE('',#851,#853,#153,.T.);
#1073=EDGE_CURVE('',#852,#854,#154,.T.);
#1074=EDGE_CURVE('',#853,#854,#502,.T.);
#1075=EDGE_CURVE('',#853,#855,#503,.T.);
#1076=EDGE_CURVE('',#854,#856,#504,.T.);
#1077=EDGE_CURVE('',#855,#856,#505,.T.);
#1078=EDGE_CURVE('',#855,#857,#155,.T.);
#1079=EDGE_CURVE('',#856,#858,#156,.T.);
#1080=EDGE_CURVE('',#857,#858,#506,.T.);
#1081=EDGE_CURVE('',#857,#859,#507,.T.);
#1082=EDGE_CURVE('',#858,#860,#508,.T.);
#1083=EDGE_CURVE('',#859,#860,#509,.T.);
#1084=EDGE_CURVE('',#859,#861,#157,.T.);
#1085=EDGE_CURVE('',#860,#862,#158,.T.);
#1086=EDGE_CURVE('',#861,#862,#510,.T.);
#1087=EDGE_CURVE('',#863,#864,#511,.T.);
#1088=EDGE_CURVE('',#863,#865,#159,.T.);
#1089=EDGE_CURVE('',#865,#866,#512,.T.);
#1090=EDGE_CURVE('',#864,#866,#160,.T.);
#1091=EDGE_CURVE('',#867,#868,#513,.T.);
#1092=EDGE_CURVE('',#867,#863,#514,.T.);
#1093=EDGE_CURVE('',#868,#864,#515,.T.);
#1094=EDGE_CURVE('',#869,#870,#516,.T.);
#1095=EDGE_CURVE('',#869,#867,#161,.T.);
#1096=EDGE_CURVE('',#870,#868,#162,.T.);
#1097=EDGE_CURVE('',#871,#872,#517,.T.);
#1098=EDGE_CURVE('',#871,#869,#518,.T.);
#1099=EDGE_CURVE('',#872,#870,#519,.T.);
#1100=EDGE_CURVE('',#873,#874,#520,.T.);
#1101=EDGE_CURVE('',#873,#871,#163,.T.);
#1102=EDGE_CURVE('',#874,#872,#164,.T.);
#1103=EDGE_CURVE('',#875,#876,#521,.T.);
#1104=EDGE_CURVE('',#875,#873,#522,.T.);
#1105=EDGE_CURVE('',#876,#874,#523,.T.);
#1106=EDGE_CURVE('',#877,#878,#524,.T.);
#1107=EDGE_CURVE('',#877,#875,#165,.T.);
#1108=EDGE_CURVE('',#878,#876,#166,.T.);
#1109=EDGE_CURVE('',#865,#877,#525,.T.);
#1110=EDGE_CURVE('',#866,#878,#526,.T.);
#1111=EDGE_CURVE('',#861,#847,#527,.T.);
#1112=EDGE_CURVE('',#862,#849,#528,.T.);
#1113=EDGE_CURVE('',#879,#880,#167,.T.);
#1114=EDGE_CURVE('',#880,#881,#529,.T.);
#1115=EDGE_CURVE('',#881,#882,#168,.T.);
#1116=EDGE_CURVE('',#882,#883,#530,.T.);
#1117=EDGE_CURVE('',#883,#884,#169,.T.);
#1118=EDGE_CURVE('',#884,#885,#531,.T.);
#1119=EDGE_CURVE('',#885,#886,#170,.T.);
#1120=EDGE_CURVE('',#886,#879,#532,.T.);
#1121=EDGE_CURVE('',#887,#888,#533,.T.);
#1122=EDGE_CURVE('',#888,#889,#171,.T.);
#1123=EDGE_CURVE('',#889,#890,#534,.T.);
#1124=EDGE_CURVE('',#890,#891,#172,.T.);
#1125=EDGE_CURVE('',#891,#892,#535,.T.);
#1126=EDGE_CURVE('',#892,#893,#173,.T.);
#1127=EDGE_CURVE('',#893,#894,#536,.T.);
#1128=EDGE_CURVE('',#894,#887,#174,.T.);
#1168=ORIENTED_EDGE('',*,*,#921,.T.);
#1169=ORIENTED_EDGE('',*,*,#922,.T.);
#1170=ORIENTED_EDGE('',*,*,#923,.F.);
#1171=ORIENTED_EDGE('',*,*,#924,.T.);
#1172=ORIENTED_EDGE('',*,*,#925,.T.);
#1173=ORIENTED_EDGE('',*,*,#926,.T.);
#1174=ORIENTED_EDGE('',*,*,#921,.F.);
#1175=ORIENTED_EDGE('',*,*,#927,.T.);
#1176=ORIENTED_EDGE('',*,*,#928,.T.);
#1177=ORIENTED_EDGE('',*,*,#929,.T.);
#1178=ORIENTED_EDGE('',*,*,#925,.F.);
#1179=ORIENTED_EDGE('',*,*,#930,.T.);
#1180=ORIENTED_EDGE('',*,*,#931,.T.);
#1181=ORIENTED_EDGE('',*,*,#932,.T.);
#1182=ORIENTED_EDGE('',*,*,#928,.F.);
#1183=ORIENTED_EDGE('',*,*,#933,.T.);
#1184=ORIENTED_EDGE('',*,*,#934,.T.);
#1185=ORIENTED_EDGE('',*,*,#935,.T.);
#1186=ORIENTED_EDGE('',*,*,#931,.F.);
#1187=ORIENTED_EDGE('',*,*,#936,.T.);
#1188=ORIENTED_EDGE('',*,*,#937,.T.);
#1189=ORIENTED_EDGE('',*,*,#938,.T.);
#1190=ORIENTED_EDGE('',*,*,#934,.F.);
#1191=ORIENTED_EDGE('',*,*,#939,.T.);
#1192=ORIENTED_EDGE('',*,*,#940,.T.);
#1193=ORIENTED_EDGE('',*,*,#941,.T.);
#1194=ORIENTED_EDGE('',*,*,#937,.F.);
#1195=ORIENTED_EDGE('',*,*,#942,.T.);
#1196=ORIENTED_EDGE('',*,*,#923,.T.);
#1197=ORIENTED_EDGE('',*,*,#943,.T.);
#1198=ORIENTED_EDGE('',*,*,#940,.F.);
#1199=ORIENTED_EDGE('',*,*,#944,.T.);
#1200=ORIENTED_EDGE('',*,*,#945,.F.);
#1201=ORIENTED_EDGE('',*,*,#946,.F.);
#1202=ORIENTED_EDGE('',*,*,#947,.F.);
#1203=ORIENTED_EDGE('',*,*,#948,.T.);
#1204=ORIENTED_EDGE('',*,*,#949,.F.);
#1205=ORIENTED_EDGE('',*,*,#948,.F.);
#1206=ORIENTED_EDGE('',*,*,#950,.F.);
#1207=ORIENTED_EDGE('',*,*,#951,.T.);
#1208=ORIENTED_EDGE('',*,*,#952,.F.);
#1209=ORIENTED_EDGE('',*,*,#951,.F.);
#1210=ORIENTED_EDGE('',*,*,#953,.T.);
#1211=ORIENTED_EDGE('',*,*,#954,.T.);
#1212=ORIENTED_EDGE('',*,*,#955,.F.);
#1213=ORIENTED_EDGE('',*,*,#954,.F.);
#1214=ORIENTED_EDGE('',*,*,#956,.F.);
#1215=ORIENTED_EDGE('',*,*,#957,.T.);
#1216=ORIENTED_EDGE('',*,*,#958,.F.);
#1217=ORIENTED_EDGE('',*,*,#957,.F.);
#1218=ORIENTED_EDGE('',*,*,#959,.F.);
#1219=ORIENTED_EDGE('',*,*,#960,.T.);
#1220=ORIENTED_EDGE('',*,*,#961,.F.);
#1221=ORIENTED_EDGE('',*,*,#960,.F.);
#1222=ORIENTED_EDGE('',*,*,#962,.F.);
#1223=ORIENTED_EDGE('',*,*,#963,.T.);
#1224=ORIENTED_EDGE('',*,*,#964,.T.);
#1225=ORIENTED_EDGE('',*,*,#963,.F.);
#1226=ORIENTED_EDGE('',*,*,#965,.F.);
#1227=ORIENTED_EDGE('',*,*,#966,.T.);
#1228=ORIENTED_EDGE('',*,*,#967,.F.);
#1229=ORIENTED_EDGE('',*,*,#966,.F.);
#1230=ORIENTED_EDGE('',*,*,#968,.F.);
#1231=ORIENTED_EDGE('',*,*,#946,.T.);
#1232=ORIENTED_EDGE('',*,*,#962,.T.);
#1233=ORIENTED_EDGE('',*,*,#959,.T.);
#1234=ORIENTED_EDGE('',*,*,#956,.T.);
#1235=ORIENTED_EDGE('',*,*,#953,.F.);
#1236=ORIENTED_EDGE('',*,*,#950,.T.);
#1237=ORIENTED_EDGE('',*,*,#947,.T.);
#1238=ORIENTED_EDGE('',*,*,#968,.T.);
#1239=ORIENTED_EDGE('',*,*,#965,.T.);
#1240=ORIENTED_EDGE('',*,*,#942,.F.);
#1241=ORIENTED_EDGE('',*,*,#939,.F.);
#1242=ORIENTED_EDGE('',*,*,#936,.F.);
#1243=ORIENTED_EDGE('',*,*,#933,.F.);
#1244=ORIENTED_EDGE('',*,*,#930,.F.);
#1245=ORIENTED_EDGE('',*,*,#927,.F.);
#1246=ORIENTED_EDGE('',*,*,#924,.F.);
#1247=ORIENTED_EDGE('',*,*,#944,.F.);
#1248=ORIENTED_EDGE('',*,*,#955,.T.);
#1249=ORIENTED_EDGE('',*,*,#958,.T.);
#1250=ORIENTED_EDGE('',*,*,#961,.T.);
#1251=ORIENTED_EDGE('',*,*,#964,.F.);
#1252=ORIENTED_EDGE('',*,*,#967,.T.);
#1253=ORIENTED_EDGE('',*,*,#945,.T.);
#1254=ORIENTED_EDGE('',*,*,#949,.T.);
#1255=ORIENTED_EDGE('',*,*,#952,.T.);
#1256=ORIENTED_EDGE('',*,*,#926,.F.);
#1257=ORIENTED_EDGE('',*,*,#929,.F.);
#1258=ORIENTED_EDGE('',*,*,#932,.F.);
#1259=ORIENTED_EDGE('',*,*,#935,.F.);
#1260=ORIENTED_EDGE('',*,*,#938,.F.);
#1261=ORIENTED_EDGE('',*,*,#941,.F.);
#1262=ORIENTED_EDGE('',*,*,#943,.F.);
#1263=ORIENTED_EDGE('',*,*,#922,.F.);
#1264=ORIENTED_EDGE('',*,*,#969,.T.);
#1265=ORIENTED_EDGE('',*,*,#970,.T.);
#1266=ORIENTED_EDGE('',*,*,#971,.F.);
#1267=ORIENTED_EDGE('',*,*,#972,.T.);
#1268=ORIENTED_EDGE('',*,*,#973,.T.);
#1269=ORIENTED_EDGE('',*,*,#974,.T.);
#1270=ORIENTED_EDGE('',*,*,#969,.F.);
#1271=ORIENTED_EDGE('',*,*,#975,.T.);
#1272=ORIENTED_EDGE('',*,*,#976,.T.);
#1273=ORIENTED_EDGE('',*,*,#977,.T.);
#1274=ORIENTED_EDGE('',*,*,#973,.F.);
#1275=ORIENTED_EDGE('',*,*,#978,.T.);
#1276=ORIENTED_EDGE('',*,*,#979,.T.);
#1277=ORIENTED_EDGE('',*,*,#980,.T.);
#1278=ORIENTED_EDGE('',*,*,#976,.F.);
#1279=ORIENTED_EDGE('',*,*,#981,.T.);
#1280=ORIENTED_EDGE('',*,*,#982,.T.);
#1281=ORIENTED_EDGE('',*,*,#983,.T.);
#1282=ORIENTED_EDGE('',*,*,#979,.F.);
#1283=ORIENTED_EDGE('',*,*,#984,.T.);
#1284=ORIENTED_EDGE('',*,*,#985,.T.);
#1285=ORIENTED_EDGE('',*,*,#986,.T.);
#1286=ORIENTED_EDGE('',*,*,#982,.F.);
#1287=ORIENTED_EDGE('',*,*,#987,.T.);
#1288=ORIENTED_EDGE('',*,*,#988,.T.);
#1289=ORIENTED_EDGE('',*,*,#989,.T.);
#1290=ORIENTED_EDGE('',*,*,#985,.F.);
#1291=ORIENTED_EDGE('',*,*,#990,.T.);
#1292=ORIENTED_EDGE('',*,*,#971,.T.);
#1293=ORIENTED_EDGE('',*,*,#991,.T.);
#1294=ORIENTED_EDGE('',*,*,#988,.F.);
#1295=ORIENTED_EDGE('',*,*,#992,.T.);
#1296=ORIENTED_EDGE('',*,*,#993,.F.);
#1297=ORIENTED_EDGE('',*,*,#994,.F.);
#1298=ORIENTED_EDGE('',*,*,#995,.F.);
#1299=ORIENTED_EDGE('',*,*,#996,.T.);
#1300=ORIENTED_EDGE('',*,*,#997,.F.);
#1301=ORIENTED_EDGE('',*,*,#996,.F.);
#1302=ORIENTED_EDGE('',*,*,#998,.F.);
#1303=ORIENTED_EDGE('',*,*,#999,.T.);
#1304=ORIENTED_EDGE('',*,*,#1000,.F.);
#1305=ORIENTED_EDGE('',*,*,#999,.F.);
#1306=ORIENTED_EDGE('',*,*,#1001,.T.);
#1307=ORIENTED_EDGE('',*,*,#1002,.T.);
#1308=ORIENTED_EDGE('',*,*,#1003,.F.);
#1309=ORIENTED_EDGE('',*,*,#1002,.F.);
#1310=ORIENTED_EDGE('',*,*,#1004,.F.);
#1311=ORIENTED_EDGE('',*,*,#1005,.T.);
#1312=ORIENTED_EDGE('',*,*,#1006,.F.);
#1313=ORIENTED_EDGE('',*,*,#1005,.F.);
#1314=ORIENTED_EDGE('',*,*,#1007,.F.);
#1315=ORIENTED_EDGE('',*,*,#1008,.T.);
#1316=ORIENTED_EDGE('',*,*,#1009,.F.);
#1317=ORIENTED_EDGE('',*,*,#1008,.F.);
#1318=ORIENTED_EDGE('',*,*,#1010,.F.);
#1319=ORIENTED_EDGE('',*,*,#1011,.T.);
#1320=ORIENTED_EDGE('',*,*,#1012,.T.);
#1321=ORIENTED_EDGE('',*,*,#1011,.F.);
#1322=ORIENTED_EDGE('',*,*,#1013,.F.);
#1323=ORIENTED_EDGE('',*,*,#1014,.T.);
#1324=ORIENTED_EDGE('',*,*,#1015,.F.);
#1325=ORIENTED_EDGE('',*,*,#1014,.F.);
#1326=ORIENTED_EDGE('',*,*,#1016,.F.);
#1327=ORIENTED_EDGE('',*,*,#994,.T.);
#1328=ORIENTED_EDGE('',*,*,#1010,.T.);
#1329=ORIENTED_EDGE('',*,*,#1007,.T.);
#1330=ORIENTED_EDGE('',*,*,#1004,.T.);
#1331=ORIENTED_EDGE('',*,*,#1001,.F.);
#1332=ORIENTED_EDGE('',*,*,#998,.T.);
#1333=ORIENTED_EDGE('',*,*,#995,.T.);
#1334=ORIENTED_EDGE('',*,*,#1016,.T.);
#1335=ORIENTED_EDGE('',*,*,#1013,.T.);
#1336=ORIENTED_EDGE('',*,*,#990,.F.);
#1337=ORIENTED_EDGE('',*,*,#987,.F.);
#1338=ORIENTED_EDGE('',*,*,#984,.F.);
#1339=ORIENTED_EDGE('',*,*,#981,.F.);
#1340=ORIENTED_EDGE('',*,*,#978,.F.);
#1341=ORIENTED_EDGE('',*,*,#975,.F.);
#1342=ORIENTED_EDGE('',*,*,#972,.F.);
#1343=ORIENTED_EDGE('',*,*,#992,.F.);
#1344=ORIENTED_EDGE('',*,*,#1003,.T.);
#1345=ORIENTED_EDGE('',*,*,#1006,.T.);
#1346=ORIENTED_EDGE('',*,*,#1009,.T.);
#1347=ORIENTED_EDGE('',*,*,#1012,.F.);
#1348=ORIENTED_EDGE('',*,*,#1015,.T.);
#1349=ORIENTED_EDGE('',*,*,#993,.T.);
#1350=ORIENTED_EDGE('',*,*,#997,.T.);
#1351=ORIENTED_EDGE('',*,*,#1000,.T.);
#1352=ORIENTED_EDGE('',*,*,#974,.F.);
#1353=ORIENTED_EDGE('',*,*,#977,.F.);
#1354=ORIENTED_EDGE('',*,*,#980,.F.);
#1355=ORIENTED_EDGE('',*,*,#983,.F.);
#1356=ORIENTED_EDGE('',*,*,#986,.F.);
#1357=ORIENTED_EDGE('',*,*,#989,.F.);
#1358=ORIENTED_EDGE('',*,*,#991,.F.);
#1359=ORIENTED_EDGE('',*,*,#970,.F.);
#1360=ORIENTED_EDGE('',*,*,#1017,.F.);
#1361=ORIENTED_EDGE('',*,*,#1018,.T.);
#1362=ORIENTED_EDGE('',*,*,#1019,.T.);
#1363=ORIENTED_EDGE('',*,*,#1020,.F.);
#1364=ORIENTED_EDGE('',*,*,#1021,.F.);
#1365=ORIENTED_EDGE('',*,*,#1020,.T.);
#1366=ORIENTED_EDGE('',*,*,#1022,.T.);
#1367=ORIENTED_EDGE('',*,*,#1023,.F.);
#1368=ORIENTED_EDGE('',*,*,#1024,.F.);
#1369=ORIENTED_EDGE('',*,*,#1023,.T.);
#1370=ORIENTED_EDGE('',*,*,#1025,.T.);
#1371=ORIENTED_EDGE('',*,*,#1026,.F.);
#1372=ORIENTED_EDGE('',*,*,#1027,.F.);
#1373=ORIENTED_EDGE('',*,*,#1026,.T.);
#1374=ORIENTED_EDGE('',*,*,#1028,.T.);
#1375=ORIENTED_EDGE('',*,*,#1029,.F.);
#1376=ORIENTED_EDGE('',*,*,#1030,.F.);
#1377=ORIENTED_EDGE('',*,*,#1029,.T.);
#1378=ORIENTED_EDGE('',*,*,#1031,.T.);
#1379=ORIENTED_EDGE('',*,*,#1032,.F.);
#1380=ORIENTED_EDGE('',*,*,#1033,.F.);
#1381=ORIENTED_EDGE('',*,*,#1032,.T.);
#1382=ORIENTED_EDGE('',*,*,#1034,.T.);
#1383=ORIENTED_EDGE('',*,*,#1035,.F.);
#1384=ORIENTED_EDGE('',*,*,#1036,.F.);
#1385=ORIENTED_EDGE('',*,*,#1035,.T.);
#1386=ORIENTED_EDGE('',*,*,#1037,.T.);
#1387=ORIENTED_EDGE('',*,*,#1038,.F.);
#1388=ORIENTED_EDGE('',*,*,#1039,.F.);
#1389=ORIENTED_EDGE('',*,*,#1040,.T.);
#1390=ORIENTED_EDGE('',*,*,#1041,.T.);
#1391=ORIENTED_EDGE('',*,*,#1042,.F.);
#1392=ORIENTED_EDGE('',*,*,#1043,.F.);
#1393=ORIENTED_EDGE('',*,*,#1044,.T.);
#1394=ORIENTED_EDGE('',*,*,#1039,.T.);
#1395=ORIENTED_EDGE('',*,*,#1045,.F.);
#1396=ORIENTED_EDGE('',*,*,#1046,.F.);
#1397=ORIENTED_EDGE('',*,*,#1047,.T.);
#1398=ORIENTED_EDGE('',*,*,#1043,.T.);
#1399=ORIENTED_EDGE('',*,*,#1048,.F.);
#1400=ORIENTED_EDGE('',*,*,#1049,.F.);
#1401=ORIENTED_EDGE('',*,*,#1050,.T.);
#1402=ORIENTED_EDGE('',*,*,#1046,.T.);
#1403=ORIENTED_EDGE('',*,*,#1051,.F.);
#1404=ORIENTED_EDGE('',*,*,#1052,.F.);
#1405=ORIENTED_EDGE('',*,*,#1053,.T.);
#1406=ORIENTED_EDGE('',*,*,#1049,.T.);
#1407=ORIENTED_EDGE('',*,*,#1054,.F.);
#1408=ORIENTED_EDGE('',*,*,#1055,.F.);
#1409=ORIENTED_EDGE('',*,*,#1056,.T.);
#1410=ORIENTED_EDGE('',*,*,#1052,.T.);
#1411=ORIENTED_EDGE('',*,*,#1057,.F.);
#1412=ORIENTED_EDGE('',*,*,#1058,.F.);
#1413=ORIENTED_EDGE('',*,*,#1059,.T.);
#1414=ORIENTED_EDGE('',*,*,#1055,.T.);
#1415=ORIENTED_EDGE('',*,*,#1060,.F.);
#1416=ORIENTED_EDGE('',*,*,#1041,.F.);
#1417=ORIENTED_EDGE('',*,*,#1061,.T.);
#1418=ORIENTED_EDGE('',*,*,#1058,.T.);
#1419=ORIENTED_EDGE('',*,*,#1062,.F.);
#1420=ORIENTED_EDGE('',*,*,#1063,.F.);
#1421=ORIENTED_EDGE('',*,*,#1038,.T.);
#1422=ORIENTED_EDGE('',*,*,#1064,.T.);
#1423=ORIENTED_EDGE('',*,*,#1018,.F.);
#1424=ORIENTED_EDGE('',*,*,#1019,.F.);
#1425=ORIENTED_EDGE('',*,*,#1064,.F.);
#1426=ORIENTED_EDGE('',*,*,#1037,.F.);
#1427=ORIENTED_EDGE('',*,*,#1034,.F.);
#1428=ORIENTED_EDGE('',*,*,#1031,.F.);
#1429=ORIENTED_EDGE('',*,*,#1028,.F.);
#1430=ORIENTED_EDGE('',*,*,#1025,.F.);
#1431=ORIENTED_EDGE('',*,*,#1022,.F.);
#1432=ORIENTED_EDGE('',*,*,#1042,.T.);
#1433=ORIENTED_EDGE('',*,*,#1062,.T.);
#1434=ORIENTED_EDGE('',*,*,#1060,.T.);
#1435=ORIENTED_EDGE('',*,*,#1057,.T.);
#1436=ORIENTED_EDGE('',*,*,#1054,.T.);
#1437=ORIENTED_EDGE('',*,*,#1051,.T.);
#1438=ORIENTED_EDGE('',*,*,#1048,.T.);
#1439=ORIENTED_EDGE('',*,*,#1045,.T.);
#1440=ORIENTED_EDGE('',*,*,#1063,.T.);
#1441=ORIENTED_EDGE('',*,*,#1017,.T.);
#1442=ORIENTED_EDGE('',*,*,#1021,.T.);
#1443=ORIENTED_EDGE('',*,*,#1024,.T.);
#1444=ORIENTED_EDGE('',*,*,#1027,.T.);
#1445=ORIENTED_EDGE('',*,*,#1030,.T.);
#1446=ORIENTED_EDGE('',*,*,#1033,.T.);
#1447=ORIENTED_EDGE('',*,*,#1036,.T.);
#1448=ORIENTED_EDGE('',*,*,#1040,.F.);
#1449=ORIENTED_EDGE('',*,*,#1044,.F.);
#1450=ORIENTED_EDGE('',*,*,#1047,.F.);
#1451=ORIENTED_EDGE('',*,*,#1050,.F.);
#1452=ORIENTED_EDGE('',*,*,#1053,.F.);
#1453=ORIENTED_EDGE('',*,*,#1056,.F.);
#1454=ORIENTED_EDGE('',*,*,#1059,.F.);
#1455=ORIENTED_EDGE('',*,*,#1061,.F.);
#1456=ORIENTED_EDGE('',*,*,#1065,.F.);
#1457=ORIENTED_EDGE('',*,*,#1066,.T.);
#1458=ORIENTED_EDGE('',*,*,#1067,.T.);
#1459=ORIENTED_EDGE('',*,*,#1068,.F.);
#1460=ORIENTED_EDGE('',*,*,#1069,.F.);
#1461=ORIENTED_EDGE('',*,*,#1068,.T.);
#1462=ORIENTED_EDGE('',*,*,#1070,.T.);
#1463=ORIENTED_EDGE('',*,*,#1071,.F.);
#1464=ORIENTED_EDGE('',*,*,#1072,.F.);
#1465=ORIENTED_EDGE('',*,*,#1071,.T.);
#1466=ORIENTED_EDGE('',*,*,#1073,.T.);
#1467=ORIENTED_EDGE('',*,*,#1074,.F.);
#1468=ORIENTED_EDGE('',*,*,#1075,.F.);
#1469=ORIENTED_EDGE('',*,*,#1074,.T.);
#1470=ORIENTED_EDGE('',*,*,#1076,.T.);
#1471=ORIENTED_EDGE('',*,*,#1077,.F.);
#1472=ORIENTED_EDGE('',*,*,#1078,.F.);
#1473=ORIENTED_EDGE('',*,*,#1077,.T.);
#1474=ORIENTED_EDGE('',*,*,#1079,.T.);
#1475=ORIENTED_EDGE('',*,*,#1080,.F.);
#1476=ORIENTED_EDGE('',*,*,#1081,.F.);
#1477=ORIENTED_EDGE('',*,*,#1080,.T.);
#1478=ORIENTED_EDGE('',*,*,#1082,.T.);
#1479=ORIENTED_EDGE('',*,*,#1083,.F.);
#1480=ORIENTED_EDGE('',*,*,#1084,.F.);
#1481=ORIENTED_EDGE('',*,*,#1083,.T.);
#1482=ORIENTED_EDGE('',*,*,#1085,.T.);
#1483=ORIENTED_EDGE('',*,*,#1086,.F.);
#1484=ORIENTED_EDGE('',*,*,#1087,.F.);
#1485=ORIENTED_EDGE('',*,*,#1088,.T.);
#1486=ORIENTED_EDGE('',*,*,#1089,.T.);
#1487=ORIENTED_EDGE('',*,*,#1090,.F.);
#1488=ORIENTED_EDGE('',*,*,#1091,.F.);
#1489=ORIENTED_EDGE('',*,*,#1092,.T.);
#1490=ORIENTED_EDGE('',*,*,#1087,.T.);
#1491=ORIENTED_EDGE('',*,*,#1093,.F.);
#1492=ORIENTED_EDGE('',*,*,#1094,.F.);
#1493=ORIENTED_EDGE('',*,*,#1095,.T.);
#1494=ORIENTED_EDGE('',*,*,#1091,.T.);
#1495=ORIENTED_EDGE('',*,*,#1096,.F.);
#1496=ORIENTED_EDGE('',*,*,#1097,.F.);
#1497=ORIENTED_EDGE('',*,*,#1098,.T.);
#1498=ORIENTED_EDGE('',*,*,#1094,.T.);
#1499=ORIENTED_EDGE('',*,*,#1099,.F.);
#1500=ORIENTED_EDGE('',*,*,#1100,.F.);
#1501=ORIENTED_EDGE('',*,*,#1101,.T.);
#1502=ORIENTED_EDGE('',*,*,#1097,.T.);
#1503=ORIENTED_EDGE('',*,*,#1102,.F.);
#1504=ORIENTED_EDGE('',*,*,#1103,.F.);
#1505=ORIENTED_EDGE('',*,*,#1104,.T.);
#1506=ORIENTED_EDGE('',*,*,#1100,.T.);
#1507=ORIENTED_EDGE('',*,*,#1105,.F.);
#1508=ORIENTED_EDGE('',*,*,#1106,.F.);
#1509=ORIENTED_EDGE('',*,*,#1107,.T.);
#1510=ORIENTED_EDGE('',*,*,#1103,.T.);
#1511=ORIENTED_EDGE('',*,*,#1108,.F.);
#1512=ORIENTED_EDGE('',*,*,#1089,.F.);
#1513=ORIENTED_EDGE('',*,*,#1109,.T.);
#1514=ORIENTED_EDGE('',*,*,#1106,.T.);
#1515=ORIENTED_EDGE('',*,*,#1110,.F.);
#1516=ORIENTED_EDGE('',*,*,#1111,.F.);
#1517=ORIENTED_EDGE('',*,*,#1086,.T.);
#1518=ORIENTED_EDGE('',*,*,#1112,.T.);
#1519=ORIENTED_EDGE('',*,*,#1066,.F.);
#1520=ORIENTED_EDGE('',*,*,#1067,.F.);
#1521=ORIENTED_EDGE('',*,*,#1112,.F.);
#1522=ORIENTED_EDGE('',*,*,#1085,.F.);
#1523=ORIENTED_EDGE('',*,*,#1082,.F.);
#1524=ORIENTED_EDGE('',*,*,#1079,.F.);
#1525=ORIENTED_EDGE('',*,*,#1076,.F.);
#1526=ORIENTED_EDGE('',*,*,#1073,.F.);
#1527=ORIENTED_EDGE('',*,*,#1070,.F.);
#1528=ORIENTED_EDGE('',*,*,#1090,.T.);
#1529=ORIENTED_EDGE('',*,*,#1110,.T.);
#1530=ORIENTED_EDGE('',*,*,#1108,.T.);
#1531=ORIENTED_EDGE('',*,*,#1105,.T.);
#1532=ORIENTED_EDGE('',*,*,#1102,.T.);
#1533=ORIENTED_EDGE('',*,*,#1099,.T.);
#1534=ORIENTED_EDGE('',*,*,#1096,.T.);
#1535=ORIENTED_EDGE('',*,*,#1093,.T.);
#1536=ORIENTED_EDGE('',*,*,#1111,.T.);
#1537=ORIENTED_EDGE('',*,*,#1065,.T.);
#1538=ORIENTED_EDGE('',*,*,#1069,.T.);
#1539=ORIENTED_EDGE('',*,*,#1072,.T.);
#1540=ORIENTED_EDGE('',*,*,#1075,.T.);
#1541=ORIENTED_EDGE('',*,*,#1078,.T.);
#1542=ORIENTED_EDGE('',*,*,#1081,.T.);
#1543=ORIENTED_EDGE('',*,*,#1084,.T.);
#1544=ORIENTED_EDGE('',*,*,#1088,.F.);
#1545=ORIENTED_EDGE('',*,*,#1092,.F.);
#1546=ORIENTED_EDGE('',*,*,#1095,.F.);
#1547=ORIENTED_EDGE('',*,*,#1098,.F.);
#1548=ORIENTED_EDGE('',*,*,#1101,.F.);
#1549=ORIENTED_EDGE('',*,*,#1104,.F.);
#1550=ORIENTED_EDGE('',*,*,#1107,.F.);
#1551=ORIENTED_EDGE('',*,*,#1109,.F.);
#1552=ORIENTED_EDGE('',*,*,#1113,.T.);
#1553=ORIENTED_EDGE('',*,*,#1114,.T.);
#1554=ORIENTED_EDGE('',*,*,#1115,.T.);
#1555=ORIENTED_EDGE('',*,*,#1116,.T.);
#1556=ORIENTED_EDGE('',*,*,#1117,.T.);
#1557=ORIENTED_EDGE('',*,*,#1118,.T.);
#1558=ORIENTED_EDGE('',*,*,#1119,.T.);
#1559=ORIENTED_EDGE('',*,*,#1120,.T.);
#1560=ORIENTED_EDGE('',*,*,#1121,.T.);
#1561=ORIENTED_EDGE('',*,*,#1122,.T.);
#1562=ORIENTED_EDGE('',*,*,#1123,.T.);
#1563=ORIENTED_EDGE('',*,*,#1124,.T.);
#1564=ORIENTED_EDGE('',*,*,#1125,.T.);
#1565=ORIENTED_EDGE('',*,*,#1126,.T.);
#1566=ORIENTED_EDGE('',*,*,#1127,.T.);
#1567=ORIENTED_EDGE('',*,*,#1128,.T.);
#1646=PLANE('',#1854);
#1647=PLANE('',#1858);
#1648=PLANE('',#1862);
#1649=PLANE('',#1866);
#1650=PLANE('',#1870);
#1651=PLANE('',#1874);
#1652=PLANE('',#1878);
#1653=PLANE('',#1882);
#1654=PLANE('',#1886);
#1655=PLANE('',#1887);
#1656=PLANE('',#1888);
#1657=PLANE('',#1892);
#1658=PLANE('',#1896);
#1659=PLANE('',#1900);
#1660=PLANE('',#1904);
#1661=PLANE('',#1908);
#1662=PLANE('',#1912);
#1663=PLANE('',#1916);
#1664=PLANE('',#1920);
#1665=PLANE('',#1921);
#1666=PLANE('',#1925);
#1667=PLANE('',#1929);
#1668=PLANE('',#1933);
#1669=PLANE('',#1940);
#1670=PLANE('',#1944);
#1671=PLANE('',#1948);
#1672=PLANE('',#1952);
#1673=PLANE('',#1953);
#1674=PLANE('',#1954);
#1675=PLANE('',#1955);
#1676=PLANE('',#1959);
#1677=PLANE('',#1963);
#1678=PLANE('',#1967);
#1679=PLANE('',#1974);
#1680=PLANE('',#1978);
#1681=PLANE('',#1982);
#1682=PLANE('',#1986);
#1683=PLANE('',#1987);
#1684=PLANE('',#1988);
#1685=PLANE('',#1989);
#1686=PLANE('',#1990);
#1687=PLANE('',#1995);
#1707=ADVANCED_FACE('',(#207),#1646,.T.);
#1708=ADVANCED_FACE('',(#208),#175,.F.);
#1709=ADVANCED_FACE('',(#209),#1647,.T.);
#1710=ADVANCED_FACE('',(#210),#176,.F.);
#1711=ADVANCED_FACE('',(#211),#1648,.T.);
#1712=ADVANCED_FACE('',(#212),#177,.F.);
#1713=ADVANCED_FACE('',(#213),#1649,.T.);
#1714=ADVANCED_FACE('',(#214),#178,.F.);
#1715=ADVANCED_FACE('',(#215),#1650,.F.);
#1716=ADVANCED_FACE('',(#216),#179,.T.);
#1717=ADVANCED_FACE('',(#217),#1651,.F.);
#1718=ADVANCED_FACE('',(#218),#180,.T.);
#1719=ADVANCED_FACE('',(#219),#1652,.F.);
#1720=ADVANCED_FACE('',(#220),#181,.T.);
#1721=ADVANCED_FACE('',(#221),#1653,.F.);
#1722=ADVANCED_FACE('',(#222),#182,.T.);
#1723=ADVANCED_FACE('',(#223,#95),#1654,.T.);
#1724=ADVANCED_FACE('',(#224,#96),#1655,.T.);
#1725=ADVANCED_FACE('',(#225),#1656,.T.);
#1726=ADVANCED_FACE('',(#226),#183,.F.);
#1727=ADVANCED_FACE('',(#227),#1657,.T.);
#1728=ADVANCED_FACE('',(#228),#184,.F.);
#1729=ADVANCED_FACE('',(#229),#1658,.T.);
#1730=ADVANCED_FACE('',(#230),#185,.F.);
#1731=ADVANCED_FACE('',(#231),#1659,.T.);
#1732=ADVANCED_FACE('',(#232),#186,.F.);
#1733=ADVANCED_FACE('',(#233),#1660,.F.);
#1734=ADVANCED_FACE('',(#234),#187,.T.);
#1735=ADVANCED_FACE('',(#235),#1661,.F.);
#1736=ADVANCED_FACE('',(#236),#188,.T.);
#1737=ADVANCED_FACE('',(#237),#1662,.F.);
#1738=ADVANCED_FACE('',(#238),#189,.T.);
#1739=ADVANCED_FACE('',(#239),#1663,.F.);
#1740=ADVANCED_FACE('',(#240),#190,.T.);
#1741=ADVANCED_FACE('',(#241,#97),#1664,.T.);
#1742=ADVANCED_FACE('',(#242,#98),#1665,.T.);
#1743=ADVANCED_FACE('',(#243),#191,.T.);
#1744=ADVANCED_FACE('',(#244),#1666,.F.);
#1745=ADVANCED_FACE('',(#245),#192,.T.);
#1746=ADVANCED_FACE('',(#246),#1667,.F.);
#1747=ADVANCED_FACE('',(#247),#193,.T.);
#1748=ADVANCED_FACE('',(#248),#1668,.F.);
#1749=ADVANCED_FACE('',(#249),#194,.T.);
#1750=ADVANCED_FACE('',(#250),#195,.F.);
#1751=ADVANCED_FACE('',(#251),#1669,.T.);
#1752=ADVANCED_FACE('',(#252),#196,.F.);
#1753=ADVANCED_FACE('',(#253),#1670,.T.);
#1754=ADVANCED_FACE('',(#254),#197,.F.);
#1755=ADVANCED_FACE('',(#255),#1671,.T.);
#1756=ADVANCED_FACE('',(#256),#198,.F.);
#1757=ADVANCED_FACE('',(#257),#1672,.T.);
#1758=ADVANCED_FACE('',(#258),#1673,.F.);
#1759=ADVANCED_FACE('',(#259,#99),#1674,.F.);
#1760=ADVANCED_FACE('',(#260,#100),#1675,.T.);
#1761=ADVANCED_FACE('',(#261),#199,.T.);
#1762=ADVANCED_FACE('',(#262),#1676,.F.);
#1763=ADVANCED_FACE('',(#263),#200,.T.);
#1764=ADVANCED_FACE('',(#264),#1677,.F.);
#1765=ADVANCED_FACE('',(#265),#201,.T.);
#1766=ADVANCED_FACE('',(#266),#1678,.F.);
#1767=ADVANCED_FACE('',(#267),#202,.T.);
#1768=ADVANCED_FACE('',(#268),#203,.F.);
#1769=ADVANCED_FACE('',(#269),#1679,.T.);
#1770=ADVANCED_FACE('',(#270),#204,.F.);
#1771=ADVANCED_FACE('',(#271),#1680,.T.);
#1772=ADVANCED_FACE('',(#272),#205,.F.);
#1773=ADVANCED_FACE('',(#273),#1681,.T.);
#1774=ADVANCED_FACE('',(#274),#206,.F.);
#1775=ADVANCED_FACE('',(#275),#1682,.T.);
#1776=ADVANCED_FACE('',(#276),#1683,.F.);
#1777=ADVANCED_FACE('',(#277,#101),#1684,.F.);
#1778=ADVANCED_FACE('',(#278,#102),#1685,.T.);
#1779=ADVANCED_FACE('',(#279),#1686,.T.);
#1780=ADVANCED_FACE('',(#280),#1687,.T.);
#1800=CLOSED_SHELL('',(#1707,#1708,#1709,#1710,#1711,#1712,#1713,#1714,
#1715,#1716,#1717,#1718,#1719,#1720,#1721,#1722,#1723,#1724));
#1801=CLOSED_SHELL('',(#1725,#1726,#1727,#1728,#1729,#1730,#1731,#1732,
#1733,#1734,#1735,#1736,#1737,#1738,#1739,#1740,#1741,#1742));
#1802=CLOSED_SHELL('',(#1743,#1744,#1745,#1746,#1747,#1748,#1749,#1750,
#1751,#1752,#1753,#1754,#1755,#1756,#1757,#1758,#1759,#1760));
#1803=CLOSED_SHELL('',(#1761,#1762,#1763,#1764,#1765,#1766,#1767,#1768,
#1769,#1770,#1771,#1772,#1773,#1774,#1775,#1776,#1777,#1778));
#1853=AXIS2_PLACEMENT_3D('',#2580,#2038,#2039);
#1854=AXIS2_PLACEMENT_3D('',#2581,#2040,#2041);
#1855=AXIS2_PLACEMENT_3D('',#2590,#2046,#2047);
#1856=AXIS2_PLACEMENT_3D('',#2594,#2049,#2050);
#1857=AXIS2_PLACEMENT_3D('',#2595,#2051,#2052);
#1858=AXIS2_PLACEMENT_3D('',#2596,#2053,#2054);
#1859=AXIS2_PLACEMENT_3D('',#2602,#2058,#2059);
#1860=AXIS2_PLACEMENT_3D('',#2606,#2061,#2062);
#1861=AXIS2_PLACEMENT_3D('',#2607,#2063,#2064);
#1862=AXIS2_PLACEMENT_3D('',#2608,#2065,#2066);
#1863=AXIS2_PLACEMENT_3D('',#2614,#2070,#2071);
#1864=AXIS2_PLACEMENT_3D('',#2618,#2073,#2074);
#1865=AXIS2_PLACEMENT_3D('',#2619,#2075,#2076);
#1866=AXIS2_PLACEMENT_3D('',#2620,#2077,#2078);
#1867=AXIS2_PLACEMENT_3D('',#2626,#2082,#2083);
#1868=AXIS2_PLACEMENT_3D('',#2627,#2084,#2085);
#1869=AXIS2_PLACEMENT_3D('',#2628,#2086,#2087);
#1870=AXIS2_PLACEMENT_3D('',#2629,#2088,#2089);
#1871=AXIS2_PLACEMENT_3D('',#2638,#2094,#2095);
#1872=AXIS2_PLACEMENT_3D('',#2640,#2096,#2097);
#1873=AXIS2_PLACEMENT_3D('',#2642,#2098,#2099);
#1874=AXIS2_PLACEMENT_3D('',#2644,#2101,#2102);
#1875=AXIS2_PLACEMENT_3D('',#2650,#2106,#2107);
#1876=AXIS2_PLACEMENT_3D('',#2652,#2108,#2109);
#1877=AXIS2_PLACEMENT_3D('',#2654,#2110,#2111);
#1878=AXIS2_PLACEMENT_3D('',#2656,#2113,#2114);
#1879=AXIS2_PLACEMENT_3D('',#2662,#2118,#2119);
#1880=AXIS2_PLACEMENT_3D('',#2664,#2120,#2121);
#1881=AXIS2_PLACEMENT_3D('',#2666,#2122,#2123);
#1882=AXIS2_PLACEMENT_3D('',#2668,#2125,#2126);
#1883=AXIS2_PLACEMENT_3D('',#2674,#2130,#2131);
#1884=AXIS2_PLACEMENT_3D('',#2675,#2132,#2133);
#1885=AXIS2_PLACEMENT_3D('',#2676,#2134,#2135);
#1886=AXIS2_PLACEMENT_3D('',#2677,#2136,#2137);
#1887=AXIS2_PLACEMENT_3D('',#2678,#2138,#2139);
#1888=AXIS2_PLACEMENT_3D('',#2679,#2140,#2141);
#1889=AXIS2_PLACEMENT_3D('',#2688,#2146,#2147);
#1890=AXIS2_PLACEMENT_3D('',#2692,#2149,#2150);
#1891=AXIS2_PLACEMENT_3D('',#2693,#2151,#2152);
#1892=AXIS2_PLACEMENT_3D('',#2694,#2153,#2154);
#1893=AXIS2_PLACEMENT_3D('',#2700,#2158,#2159);
#1894=AXIS2_PLACEMENT_3D('',#2704,#2161,#2162);
#1895=AXIS2_PLACEMENT_3D('',#2705,#2163,#2164);
#1896=AXIS2_PLACEMENT_3D('',#2706,#2165,#2166);
#1897=AXIS2_PLACEMENT_3D('',#2712,#2170,#2171);
#1898=AXIS2_PLACEMENT_3D('',#2716,#2173,#2174);
#1899=AXIS2_PLACEMENT_3D('',#2717,#2175,#2176);
#1900=AXIS2_PLACEMENT_3D('',#2718,#2177,#2178);
#1901=AXIS2_PLACEMENT_3D('',#2724,#2182,#2183);
#1902=AXIS2_PLACEMENT_3D('',#2725,#2184,#2185);
#1903=AXIS2_PLACEMENT_3D('',#2726,#2186,#2187);
#1904=AXIS2_PLACEMENT_3D('',#2727,#2188,#2189);
#1905=AXIS2_PLACEMENT_3D('',#2736,#2194,#2195);
#1906=AXIS2_PLACEMENT_3D('',#2738,#2196,#2197);
#1907=AXIS2_PLACEMENT_3D('',#2740,#2198,#2199);
#1908=AXIS2_PLACEMENT_3D('',#2742,#2201,#2202);
#1909=AXIS2_PLACEMENT_3D('',#2748,#2206,#2207);
#1910=AXIS2_PLACEMENT_3D('',#2750,#2208,#2209);
#1911=AXIS2_PLACEMENT_3D('',#2752,#2210,#2211);
#1912=AXIS2_PLACEMENT_3D('',#2754,#2213,#2214);
#1913=AXIS2_PLACEMENT_3D('',#2760,#2218,#2219);
#1914=AXIS2_PLACEMENT_3D('',#2762,#2220,#2221);
#1915=AXIS2_PLACEMENT_3D('',#2764,#2222,#2223);
#1916=AXIS2_PLACEMENT_3D('',#2766,#2225,#2226);
#1917=AXIS2_PLACEMENT_3D('',#2772,#2230,#2231);
#1918=AXIS2_PLACEMENT_3D('',#2773,#2232,#2233);
#1919=AXIS2_PLACEMENT_3D('',#2774,#2234,#2235);
#1920=AXIS2_PLACEMENT_3D('',#2775,#2236,#2237);
#1921=AXIS2_PLACEMENT_3D('',#2776,#2238,#2239);
#1922=AXIS2_PLACEMENT_3D('',#2777,#2240,#2241);
#1923=AXIS2_PLACEMENT_3D('',#2780,#2242,#2243);
#1924=AXIS2_PLACEMENT_3D('',#2784,#2245,#2246);
#1925=AXIS2_PLACEMENT_3D('',#2786,#2248,#2249);
#1926=AXIS2_PLACEMENT_3D('',#2792,#2253,#2254);
#1927=AXIS2_PLACEMENT_3D('',#2794,#2255,#2256);
#1928=AXIS2_PLACEMENT_3D('',#2796,#2257,#2258);
#1929=AXIS2_PLACEMENT_3D('',#2798,#2260,#2261);
#1930=AXIS2_PLACEMENT_3D('',#2804,#2265,#2266);
#1931=AXIS2_PLACEMENT_3D('',#2806,#2267,#2268);
#1932=AXIS2_PLACEMENT_3D('',#2808,#2269,#2270);
#1933=AXIS2_PLACEMENT_3D('',#2810,#2272,#2273);
#1934=AXIS2_PLACEMENT_3D('',#2816,#2277,#2278);
#1935=AXIS2_PLACEMENT_3D('',#2818,#2279,#2280);
#1936=AXIS2_PLACEMENT_3D('',#2820,#2281,#2282);
#1937=AXIS2_PLACEMENT_3D('',#2822,#2284,#2285);
#1938=AXIS2_PLACEMENT_3D('',#2827,#2287,#2288);
#1939=AXIS2_PLACEMENT_3D('',#2830,#2290,#2291);
#1940=AXIS2_PLACEMENT_3D('',#2831,#2292,#2293);
#1941=AXIS2_PLACEMENT_3D('',#2837,#2297,#2298);
#1942=AXIS2_PLACEMENT_3D('',#2841,#2300,#2301);
#1943=AXIS2_PLACEMENT_3D('',#2842,#2302,#2303);
#1944=AXIS2_PLACEMENT_3D('',#2843,#2304,#2305);
#1945=AXIS2_PLACEMENT_3D('',#2849,#2309,#2310);
#1946=AXIS2_PLACEMENT_3D('',#2853,#2312,#2313);
#1947=AXIS2_PLACEMENT_3D('',#2854,#2314,#2315);
#1948=AXIS2_PLACEMENT_3D('',#2855,#2316,#2317);
#1949=AXIS2_PLACEMENT_3D('',#2861,#2321,#2322);
#1950=AXIS2_PLACEMENT_3D('',#2865,#2324,#2325);
#1951=AXIS2_PLACEMENT_3D('',#2866,#2326,#2327);
#1952=AXIS2_PLACEMENT_3D('',#2867,#2328,#2329);
#1953=AXIS2_PLACEMENT_3D('',#2870,#2332,#2333);
#1954=AXIS2_PLACEMENT_3D('',#2873,#2336,#2337);
#1955=AXIS2_PLACEMENT_3D('',#2874,#2338,#2339);
#1956=AXIS2_PLACEMENT_3D('',#2875,#2340,#2341);
#1957=AXIS2_PLACEMENT_3D('',#2878,#2342,#2343);
#1958=AXIS2_PLACEMENT_3D('',#2882,#2345,#2346);
#1959=AXIS2_PLACEMENT_3D('',#2884,#2348,#2349);
#1960=AXIS2_PLACEMENT_3D('',#2890,#2353,#2354);
#1961=AXIS2_PLACEMENT_3D('',#2892,#2355,#2356);
#1962=AXIS2_PLACEMENT_3D('',#2894,#2357,#2358);
#1963=AXIS2_PLACEMENT_3D('',#2896,#2360,#2361);
#1964=AXIS2_PLACEMENT_3D('',#2902,#2365,#2366);
#1965=AXIS2_PLACEMENT_3D('',#2904,#2367,#2368);
#1966=AXIS2_PLACEMENT_3D('',#2906,#2369,#2370);
#1967=AXIS2_PLACEMENT_3D('',#2908,#2372,#2373);
#1968=AXIS2_PLACEMENT_3D('',#2914,#2377,#2378);
#1969=AXIS2_PLACEMENT_3D('',#2916,#2379,#2380);
#1970=AXIS2_PLACEMENT_3D('',#2918,#2381,#2382);
#1971=AXIS2_PLACEMENT_3D('',#2920,#2384,#2385);
#1972=AXIS2_PLACEMENT_3D('',#2925,#2387,#2388);
#1973=AXIS2_PLACEMENT_3D('',#2928,#2390,#2391);
#1974=AXIS2_PLACEMENT_3D('',#2929,#2392,#2393);
#1975=AXIS2_PLACEMENT_3D('',#2935,#2397,#2398);
#1976=AXIS2_PLACEMENT_3D('',#2939,#2400,#2401);
#1977=AXIS2_PLACEMENT_3D('',#2940,#2402,#2403);
#1978=AXIS2_PLACEMENT_3D('',#2941,#2404,#2405);
#1979=AXIS2_PLACEMENT_3D('',#2947,#2409,#2410);
#1980=AXIS2_PLACEMENT_3D('',#2951,#2412,#2413);
#1981=AXIS2_PLACEMENT_3D('',#2952,#2414,#2415);
#1982=AXIS2_PLACEMENT_3D('',#2953,#2416,#2417);
#1983=AXIS2_PLACEMENT_3D('',#2959,#2421,#2422);
#1984=AXIS2_PLACEMENT_3D('',#2963,#2424,#2425);
#1985=AXIS2_PLACEMENT_3D('',#2964,#2426,#2427);
#1986=AXIS2_PLACEMENT_3D('',#2965,#2428,#2429);
#1987=AXIS2_PLACEMENT_3D('',#2968,#2432,#2433);
#1988=AXIS2_PLACEMENT_3D('',#2971,#2436,#2437);
#1989=AXIS2_PLACEMENT_3D('',#2972,#2438,#2439);
#1990=AXIS2_PLACEMENT_3D('',#2973,#2440,#2441);
#1991=AXIS2_PLACEMENT_3D('',#2976,#2442,#2443);
#1992=AXIS2_PLACEMENT_3D('',#2980,#2445,#2446);
#1993=AXIS2_PLACEMENT_3D('',#2984,#2448,#2449);
#1994=AXIS2_PLACEMENT_3D('',#2988,#2451,#2452);
#1995=AXIS2_PLACEMENT_3D('',#2990,#2454,#2455);
#1996=AXIS2_PLACEMENT_3D('',#2995,#2457,#2458);
#1997=AXIS2_PLACEMENT_3D('',#2999,#2460,#2461);
#1998=AXIS2_PLACEMENT_3D('',#3003,#2463,#2464);
#1999=AXIS2_PLACEMENT_3D('',#3006,#2466,#2467);
#2038=DIRECTION('axis',(0.,0.,1.));
#2039=DIRECTION('refdir',(1.,0.,0.));
#2040=DIRECTION('center_axis',(1.,0.,0.));
#2041=DIRECTION('ref_axis',(0.,0.,-1.));
#2042=DIRECTION('',(0.,-1.,0.));
#2043=DIRECTION('',(0.,0.,-1.));
#2044=DIRECTION('',(0.,-1.,0.));
#2045=DIRECTION('',(0.,0.,1.));
#2046=DIRECTION('center_axis',(0.,-1.,0.));
#2047=DIRECTION('ref_axis',(0.,0.,-1.));
#2048=DIRECTION('',(0.,-1.,0.));
#2049=DIRECTION('center_axis',(0.,-1.,0.));
#2050=DIRECTION('ref_axis',(0.,0.,-1.));
#2051=DIRECTION('center_axis',(0.,1.,0.));
#2052=DIRECTION('ref_axis',(0.,0.,1.));
#2053=DIRECTION('center_axis',(0.,0.,-1.));
#2054=DIRECTION('ref_axis',(-1.,0.,0.));
#2055=DIRECTION('',(0.,-1.,0.));
#2056=DIRECTION('',(-1.,0.,0.));
#2057=DIRECTION('',(1.,0.,0.));
#2058=DIRECTION('center_axis',(0.,-1.,0.));
#2059=DIRECTION('ref_axis',(0.,0.,-1.));
#2060=DIRECTION('',(0.,-1.,0.));
#2061=DIRECTION('center_axis',(0.,-1.,0.));
#2062=DIRECTION('ref_axis',(0.,0.,-1.));
#2063=DIRECTION('center_axis',(0.,1.,0.));
#2064=DIRECTION('ref_axis',(0.,0.,1.));
#2065=DIRECTION('center_axis',(-1.,0.,0.));
#2066=DIRECTION('ref_axis',(0.,0.,1.));
#2067=DIRECTION('',(0.,-1.,0.));
#2068=DIRECTION('',(0.,0.,1.));
#2069=DIRECTION('',(0.,0.,-1.));
#2070=DIRECTION('center_axis',(0.,-1.,0.));
#2071=DIRECTION('ref_axis',(0.,0.,-1.));
#2072=DIRECTION('',(0.,-1.,0.));
#2073=DIRECTION('center_axis',(0.,-1.,0.));
#2074=DIRECTION('ref_axis',(0.,0.,-1.));
#2075=DIRECTION('center_axis',(0.,1.,0.));
#2076=DIRECTION('ref_axis',(0.,0.,1.));
#2077=DIRECTION('center_axis',(0.,0.,1.));
#2078=DIRECTION('ref_axis',(1.,0.,0.));
#2079=DIRECTION('',(0.,-1.,0.));
#2080=DIRECTION('',(1.,0.,0.));
#2081=DIRECTION('',(-1.,0.,0.));
#2082=DIRECTION('center_axis',(0.,-1.,0.));
#2083=DIRECTION('ref_axis',(0.,0.,-1.));
#2084=DIRECTION('center_axis',(0.,-1.,0.));
#2085=DIRECTION('ref_axis',(0.,0.,-1.));
#2086=DIRECTION('center_axis',(0.,1.,0.));
#2087=DIRECTION('ref_axis',(0.,0.,1.));
#2088=DIRECTION('center_axis',(-1.,0.,0.));
#2089=DIRECTION('ref_axis',(0.,0.,1.));
#2090=DIRECTION('',(0.,0.,1.));
#2091=DIRECTION('',(0.,-1.,0.));
#2092=DIRECTION('',(0.,0.,-1.));
#2093=DIRECTION('',(0.,-1.,0.));
#2094=DIRECTION('center_axis',(0.,-1.,0.));
#2095=DIRECTION('ref_axis',(0.,0.,-1.));
#2096=DIRECTION('center_axis',(0.,-1.,0.));
#2097=DIRECTION('ref_axis',(0.,0.,-1.));
#2098=DIRECTION('center_axis',(0.,1.,0.));
#2099=DIRECTION('ref_axis',(0.,0.,1.));
#2100=DIRECTION('',(0.,-1.,0.));
#2101=DIRECTION('center_axis',(0.,0.,-1.));
#2102=DIRECTION('ref_axis',(-1.,0.,0.));
#2103=DIRECTION('',(-1.,0.,0.));
#2104=DIRECTION('',(-1.,0.,0.));
#2105=DIRECTION('',(0.,-1.,0.));
#2106=DIRECTION('center_axis',(0.,-1.,0.));
#2107=DIRECTION('ref_axis',(0.,0.,-1.));
#2108=DIRECTION('center_axis',(0.,-1.,0.));
#2109=DIRECTION('ref_axis',(0.,0.,-1.));
#2110=DIRECTION('center_axis',(0.,1.,0.));
#2111=DIRECTION('ref_axis',(0.,0.,1.));
#2112=DIRECTION('',(0.,-1.,0.));
#2113=DIRECTION('center_axis',(1.,0.,0.));
#2114=DIRECTION('ref_axis',(0.,0.,-1.));
#2115=DIRECTION('',(0.,0.,-1.));
#2116=DIRECTION('',(0.,0.,1.));
#2117=DIRECTION('',(0.,-1.,0.));
#2118=DIRECTION('center_axis',(0.,-1.,0.));
#2119=DIRECTION('ref_axis',(0.,0.,-1.));
#2120=DIRECTION('center_axis',(0.,-1.,0.));
#2121=DIRECTION('ref_axis',(0.,0.,-1.));
#2122=DIRECTION('center_axis',(0.,1.,0.));
#2123=DIRECTION('ref_axis',(0.,0.,1.));
#2124=DIRECTION('',(0.,-1.,0.));
#2125=DIRECTION('center_axis',(0.,0.,1.));
#2126=DIRECTION('ref_axis',(1.,0.,0.));
#2127=DIRECTION('',(-1.,0.,0.));
#2128=DIRECTION('',(-1.,0.,0.));
#2129=DIRECTION('',(0.,-1.,0.));
#2130=DIRECTION('center_axis',(0.,-1.,0.));
#2131=DIRECTION('ref_axis',(0.,0.,-1.));
#2132=DIRECTION('center_axis',(0.,-1.,0.));
#2133=DIRECTION('ref_axis',(0.,0.,-1.));
#2134=DIRECTION('center_axis',(0.,1.,0.));
#2135=DIRECTION('ref_axis',(0.,0.,1.));
#2136=DIRECTION('center_axis',(0.,1.,0.));
#2137=DIRECTION('ref_axis',(0.,0.,1.));
#2138=DIRECTION('center_axis',(0.,-1.,0.));
#2139=DIRECTION('ref_axis',(0.,0.,-1.));
#2140=DIRECTION('center_axis',(1.,0.,0.));
#2141=DIRECTION('ref_axis',(0.,0.,-1.));
#2142=DIRECTION('',(0.,-1.,0.));
#2143=DIRECTION('',(0.,0.,-1.));
#2144=DIRECTION('',(0.,-1.,0.));
#2145=DIRECTION('',(0.,0.,1.));
#2146=DIRECTION('center_axis',(0.,-1.,0.));
#2147=DIRECTION('ref_axis',(0.,0.,-1.));
#2148=DIRECTION('',(0.,-1.,0.));
#2149=DIRECTION('center_axis',(0.,-1.,0.));
#2150=DIRECTION('ref_axis',(0.,0.,-1.));
#2151=DIRECTION('center_axis',(0.,1.,0.));
#2152=DIRECTION('ref_axis',(0.,0.,1.));
#2153=DIRECTION('center_axis',(0.,0.,-1.));
#2154=DIRECTION('ref_axis',(-1.,0.,0.));
#2155=DIRECTION('',(0.,-1.,0.));
#2156=DIRECTION('',(-1.,0.,0.));
#2157=DIRECTION('',(1.,0.,0.));
#2158=DIRECTION('center_axis',(0.,-1.,0.));
#2159=DIRECTION('ref_axis',(0.,0.,-1.));
#2160=DIRECTION('',(0.,-1.,0.));
#2161=DIRECTION('center_axis',(0.,-1.,0.));
#2162=DIRECTION('ref_axis',(0.,0.,-1.));
#2163=DIRECTION('center_axis',(0.,1.,0.));
#2164=DIRECTION('ref_axis',(0.,0.,1.));
#2165=DIRECTION('center_axis',(-1.,0.,0.));
#2166=DIRECTION('ref_axis',(0.,0.,1.));
#2167=DIRECTION('',(0.,-1.,0.));
#2168=DIRECTION('',(0.,0.,1.));
#2169=DIRECTION('',(0.,0.,-1.));
#2170=DIRECTION('center_axis',(0.,-1.,0.));
#2171=DIRECTION('ref_axis',(0.,0.,-1.));
#2172=DIRECTION('',(0.,-1.,0.));
#2173=DIRECTION('center_axis',(0.,-1.,0.));
#2174=DIRECTION('ref_axis',(0.,0.,-1.));
#2175=DIRECTION('center_axis',(0.,1.,0.));
#2176=DIRECTION('ref_axis',(0.,0.,1.));
#2177=DIRECTION('center_axis',(0.,0.,1.));
#2178=DIRECTION('ref_axis',(1.,0.,0.));
#2179=DIRECTION('',(0.,-1.,0.));
#2180=DIRECTION('',(1.,0.,0.));
#2181=DIRECTION('',(-1.,0.,0.));
#2182=DIRECTION('center_axis',(0.,-1.,0.));
#2183=DIRECTION('ref_axis',(0.,0.,-1.));
#2184=DIRECTION('center_axis',(0.,-1.,0.));
#2185=DIRECTION('ref_axis',(0.,0.,-1.));
#2186=DIRECTION('center_axis',(0.,1.,0.));
#2187=DIRECTION('ref_axis',(0.,0.,1.));
#2188=DIRECTION('center_axis',(-1.,0.,0.));
#2189=DIRECTION('ref_axis',(0.,0.,1.));
#2190=DIRECTION('',(0.,0.,1.));
#2191=DIRECTION('',(0.,-1.,0.));
#2192=DIRECTION('',(0.,0.,-1.));
#2193=DIRECTION('',(0.,-1.,0.));
#2194=DIRECTION('center_axis',(0.,-1.,0.));
#2195=DIRECTION('ref_axis',(0.,0.,-1.));
#2196=DIRECTION('center_axis',(0.,-1.,0.));
#2197=DIRECTION('ref_axis',(0.,0.,-1.));
#2198=DIRECTION('center_axis',(0.,1.,0.));
#2199=DIRECTION('ref_axis',(0.,0.,1.));
#2200=DIRECTION('',(0.,-1.,0.));
#2201=DIRECTION('center_axis',(0.,0.,-1.));
#2202=DIRECTION('ref_axis',(-1.,0.,0.));
#2203=DIRECTION('',(-1.,0.,0.));
#2204=DIRECTION('',(-1.,0.,0.));
#2205=DIRECTION('',(0.,-1.,0.));
#2206=DIRECTION('center_axis',(0.,-1.,0.));
#2207=DIRECTION('ref_axis',(0.,0.,-1.));
#2208=DIRECTION('center_axis',(0.,-1.,0.));
#2209=DIRECTION('ref_axis',(0.,0.,-1.));
#2210=DIRECTION('center_axis',(0.,1.,0.));
#2211=DIRECTION('ref_axis',(0.,0.,1.));
#2212=DIRECTION('',(0.,-1.,0.));
#2213=DIRECTION('center_axis',(1.,0.,0.));
#2214=DIRECTION('ref_axis',(0.,0.,-1.));
#2215=DIRECTION('',(0.,0.,-1.));
#2216=DIRECTION('',(0.,0.,1.));
#2217=DIRECTION('',(0.,-1.,0.));
#2218=DIRECTION('center_axis',(0.,-1.,0.));
#2219=DIRECTION('ref_axis',(0.,0.,-1.));
#2220=DIRECTION('center_axis',(0.,-1.,0.));
#2221=DIRECTION('ref_axis',(0.,0.,-1.));
#2222=DIRECTION('center_axis',(0.,1.,0.));
#2223=DIRECTION('ref_axis',(0.,0.,1.));
#2224=DIRECTION('',(0.,-1.,0.));
#2225=DIRECTION('center_axis',(0.,0.,1.));
#2226=DIRECTION('ref_axis',(1.,0.,0.));
#2227=DIRECTION('',(-1.,0.,0.));
#2228=DIRECTION('',(-1.,0.,0.));
#2229=DIRECTION('',(0.,-1.,0.));
#2230=DIRECTION('center_axis',(0.,-1.,0.));
#2231=DIRECTION('ref_axis',(0.,0.,-1.));
#2232=DIRECTION('center_axis',(0.,-1.,0.));
#2233=DIRECTION('ref_axis',(0.,0.,-1.));
#2234=DIRECTION('center_axis',(0.,1.,0.));
#2235=DIRECTION('ref_axis',(0.,0.,1.));
#2236=DIRECTION('center_axis',(0.,1.,0.));
#2237=DIRECTION('ref_axis',(0.,0.,1.));
#2238=DIRECTION('center_axis',(0.,-1.,0.));
#2239=DIRECTION('ref_axis',(0.,0.,-1.));
#2240=DIRECTION('center_axis',(-1.,0.,1.29165007961917E-51));
#2241=DIRECTION('ref_axis',(1.29165007961917E-51,0.,1.));
#2242=DIRECTION('center_axis',(1.,0.,-1.29165007961917E-51));
#2243=DIRECTION('ref_axis',(-1.29165007961917E-51,0.,-1.));
#2244=DIRECTION('',(-1.,0.,1.29165007961917E-51));
#2245=DIRECTION('center_axis',(1.,0.,-1.29165007961917E-51));
#2246=DIRECTION('ref_axis',(-1.29165007961917E-51,0.,-1.));
#2247=DIRECTION('',(-1.,0.,1.29165007961917E-51));
#2248=DIRECTION('center_axis',(-1.29165007961917E-51,0.,-1.));
#2249=DIRECTION('ref_axis',(-1.,0.,1.29165007961917E-51));
#2250=DIRECTION('',(0.,-1.,0.));
#2251=DIRECTION('',(0.,-1.,0.));
#2252=DIRECTION('',(-1.,0.,1.29165007961917E-51));
#2253=DIRECTION('center_axis',(-1.,0.,1.29165007961917E-51));
#2254=DIRECTION('ref_axis',(1.29165007961917E-51,0.,1.));
#2255=DIRECTION('center_axis',(1.,0.,-1.29165007961917E-51));
#2256=DIRECTION('ref_axis',(-1.29165007961917E-51,0.,-1.));
#2257=DIRECTION('center_axis',(1.,0.,-1.29165007961917E-51));
#2258=DIRECTION('ref_axis',(-1.29165007961917E-51,0.,-1.));
#2259=DIRECTION('',(-1.,0.,1.29165007961917E-51));
#2260=DIRECTION('center_axis',(0.,1.,0.));
#2261=DIRECTION('ref_axis',(-1.29165007961917E-51,0.,1.));
#2262=DIRECTION('',(1.29165007961917E-51,0.,-1.));
#2263=DIRECTION('',(1.29165007961917E-51,0.,-1.));
#2264=DIRECTION('',(-1.,0.,1.29165007961917E-51));
#2265=DIRECTION('center_axis',(-1.,0.,1.29165007961917E-51));
#2266=DIRECTION('ref_axis',(1.29165007961917E-51,0.,1.));
#2267=DIRECTION('center_axis',(1.,0.,-1.29165007961917E-51));
#2268=DIRECTION('ref_axis',(-1.29165007961917E-51,0.,-1.));
#2269=DIRECTION('center_axis',(1.,0.,-1.29165007961917E-51));
#2270=DIRECTION('ref_axis',(-1.29165007961917E-51,0.,-1.));
#2271=DIRECTION('',(-1.,0.,1.29165007961917E-51));
#2272=DIRECTION('center_axis',(1.29165007961917E-51,0.,1.));
#2273=DIRECTION('ref_axis',(1.,0.,-1.29165007961917E-51));
#2274=DIRECTION('',(0.,1.,0.));
#2275=DIRECTION('',(0.,1.,0.));
#2276=DIRECTION('',(-1.,0.,1.29165007961917E-51));
#2277=DIRECTION('center_axis',(-1.,0.,1.29165007961917E-51));
#2278=DIRECTION('ref_axis',(1.29165007961917E-51,0.,1.));
#2279=DIRECTION('center_axis',(1.,0.,-1.29165007961917E-51));
#2280=DIRECTION('ref_axis',(-1.29165007961917E-51,0.,-1.));
#2281=DIRECTION('center_axis',(1.,0.,-1.29165007961917E-51));
#2282=DIRECTION('ref_axis',(-1.29165007961917E-51,0.,-1.));
#2283=DIRECTION('',(-1.,0.,1.29165007961917E-51));
#2284=DIRECTION('center_axis',(-1.,0.,1.29165007961917E-51));
#2285=DIRECTION('ref_axis',(1.29165007961917E-51,0.,1.));
#2286=DIRECTION('',(-1.,0.,1.29165007961917E-51));
#2287=DIRECTION('center_axis',(1.,0.,-1.29165007961917E-51));
#2288=DIRECTION('ref_axis',(-1.29165007961917E-51,0.,-1.));
#2289=DIRECTION('',(-1.,0.,1.29165007961917E-51));
#2290=DIRECTION('center_axis',(1.,0.,-1.29165007961917E-51));
#2291=DIRECTION('ref_axis',(-1.29165007961917E-51,0.,-1.));
#2292=DIRECTION('center_axis',(-1.29165007961917E-51,0.,-1.));
#2293=DIRECTION('ref_axis',(-1.,0.,1.29165007961917E-51));
#2294=DIRECTION('',(-1.,0.,1.29165007961917E-51));
#2295=DIRECTION('',(0.,-1.,0.));
#2296=DIRECTION('',(0.,-1.,0.));
#2297=DIRECTION('center_axis',(-1.,0.,1.29165007961917E-51));
#2298=DIRECTION('ref_axis',(1.29165007961917E-51,0.,1.));
#2299=DIRECTION('',(-1.,0.,1.29165007961917E-51));
#2300=DIRECTION('center_axis',(1.,0.,-1.29165007961917E-51));
#2301=DIRECTION('ref_axis',(-1.29165007961917E-51,0.,-1.));
#2302=DIRECTION('center_axis',(1.,0.,-1.29165007961917E-51));
#2303=DIRECTION('ref_axis',(-1.29165007961917E-51,0.,-1.));
#2304=DIRECTION('center_axis',(0.,-1.,0.));
#2305=DIRECTION('ref_axis',(1.29165007961917E-51,0.,-1.));
#2306=DIRECTION('',(-1.,0.,1.29165007961917E-51));
#2307=DIRECTION('',(-1.29165007961917E-51,0.,1.));
#2308=DIRECTION('',(-1.29165007961917E-51,0.,1.));
#2309=DIRECTION('center_axis',(-1.,0.,1.29165007961917E-51));
#2310=DIRECTION('ref_axis',(1.29165007961917E-51,0.,1.));
#2311=DIRECTION('',(-1.,0.,1.29165007961917E-51));
#2312=DIRECTION('center_axis',(1.,0.,-1.29165007961917E-51));
#2313=DIRECTION('ref_axis',(-1.29165007961917E-51,0.,-1.));
#2314=DIRECTION('center_axis',(1.,0.,-1.29165007961917E-51));
#2315=DIRECTION('ref_axis',(-1.29165007961917E-51,0.,-1.));
#2316=DIRECTION('center_axis',(1.29165007961917E-51,0.,1.));
#2317=DIRECTION('ref_axis',(1.,0.,-1.29165007961917E-51));
#2318=DIRECTION('',(-1.,0.,1.29165007961917E-51));
#2319=DIRECTION('',(0.,1.,0.));
#2320=DIRECTION('',(0.,1.,0.));
#2321=DIRECTION('center_axis',(-1.,0.,1.29165007961917E-51));
#2322=DIRECTION('ref_axis',(1.29165007961917E-51,0.,1.));
#2323=DIRECTION('',(-1.,0.,1.29165007961917E-51));
#2324=DIRECTION('center_axis',(1.,0.,-1.29165007961917E-51));
#2325=DIRECTION('ref_axis',(-1.29165007961917E-51,0.,-1.));
#2326=DIRECTION('center_axis',(1.,0.,-1.29165007961917E-51));
#2327=DIRECTION('ref_axis',(-1.29165007961917E-51,0.,-1.));
#2328=DIRECTION('center_axis',(0.,1.,0.));
#2329=DIRECTION('ref_axis',(-1.29165007961917E-51,0.,1.));
#2330=DIRECTION('',(1.29165007961917E-51,0.,-1.));
#2331=DIRECTION('',(1.29165007961917E-51,0.,-1.));
#2332=DIRECTION('center_axis',(0.,-1.,0.));
#2333=DIRECTION('ref_axis',(1.29165007961917E-51,0.,-1.));
#2334=DIRECTION('',(-1.29165007961917E-51,0.,1.));
#2335=DIRECTION('',(-1.29165007961917E-51,0.,1.));
#2336=DIRECTION('center_axis',(1.,0.,1.29165007961917E-51));
#2337=DIRECTION('ref_axis',(1.29165007961917E-51,0.,-1.));
#2338=DIRECTION('center_axis',(1.,0.,1.29165007961917E-51));
#2339=DIRECTION('ref_axis',(1.29165007961917E-51,0.,-1.));
#2340=DIRECTION('center_axis',(-1.,0.,1.58362419671978E-50));
#2341=DIRECTION('ref_axis',(1.58362419671978E-50,0.,1.));
#2342=DIRECTION('center_axis',(1.,0.,-1.58362419671978E-50));
#2343=DIRECTION('ref_axis',(-1.58362419671978E-50,0.,-1.));
#2344=DIRECTION('',(-1.,0.,1.58362419671978E-50));
#2345=DIRECTION('center_axis',(1.,0.,-1.58362419671978E-50));
#2346=DIRECTION('ref_axis',(-1.58362419671978E-50,0.,-1.));
#2347=DIRECTION('',(-1.,0.,1.58362419671978E-50));
#2348=DIRECTION('center_axis',(-1.58362419671978E-50,0.,-1.));
#2349=DIRECTION('ref_axis',(-1.,0.,1.58362419671978E-50));
#2350=DIRECTION('',(0.,-1.,0.));
#2351=DIRECTION('',(0.,-1.,0.));
#2352=DIRECTION('',(-1.,0.,1.58362419671978E-50));
#2353=DIRECTION('center_axis',(-1.,0.,1.58362419671978E-50));
#2354=DIRECTION('ref_axis',(1.58362419671978E-50,0.,1.));
#2355=DIRECTION('center_axis',(1.,0.,-1.58362419671978E-50));
#2356=DIRECTION('ref_axis',(-1.58362419671978E-50,0.,-1.));
#2357=DIRECTION('center_axis',(1.,0.,-1.58362419671978E-50));
#2358=DIRECTION('ref_axis',(-1.58362419671978E-50,0.,-1.));
#2359=DIRECTION('',(-1.,0.,1.58362419671978E-50));
#2360=DIRECTION('center_axis',(0.,1.,0.));
#2361=DIRECTION('ref_axis',(-1.58362419671978E-50,0.,1.));
#2362=DIRECTION('',(1.58362419671978E-50,0.,-1.));
#2363=DIRECTION('',(1.58362419671978E-50,0.,-1.));
#2364=DIRECTION('',(-1.,0.,1.58362419671978E-50));
#2365=DIRECTION('center_axis',(-1.,0.,1.58362419671978E-50));
#2366=DIRECTION('ref_axis',(1.58362419671978E-50,0.,1.));
#2367=DIRECTION('center_axis',(1.,0.,-1.58362419671978E-50));
#2368=DIRECTION('ref_axis',(-1.58362419671978E-50,0.,-1.));
#2369=DIRECTION('center_axis',(1.,0.,-1.58362419671978E-50));
#2370=DIRECTION('ref_axis',(-1.58362419671978E-50,0.,-1.));
#2371=DIRECTION('',(-1.,0.,1.58362419671978E-50));
#2372=DIRECTION('center_axis',(1.58362419671978E-50,0.,1.));
#2373=DIRECTION('ref_axis',(1.,0.,-1.58362419671978E-50));
#2374=DIRECTION('',(0.,1.,0.));
#2375=DIRECTION('',(0.,1.,0.));
#2376=DIRECTION('',(-1.,0.,1.58362419671978E-50));
#2377=DIRECTION('center_axis',(-1.,0.,1.58362419671978E-50));
#2378=DIRECTION('ref_axis',(1.58362419671978E-50,0.,1.));
#2379=DIRECTION('center_axis',(1.,0.,-1.58362419671978E-50));
#2380=DIRECTION('ref_axis',(-1.58362419671978E-50,0.,-1.));
#2381=DIRECTION('center_axis',(1.,0.,-1.58362419671978E-50));
#2382=DIRECTION('ref_axis',(-1.58362419671978E-50,0.,-1.));
#2383=DIRECTION('',(-1.,0.,1.58362419671978E-50));
#2384=DIRECTION('center_axis',(-1.,0.,1.58362419671978E-50));
#2385=DIRECTION('ref_axis',(1.58362419671978E-50,0.,1.));
#2386=DIRECTION('',(-1.,0.,1.58362419671978E-50));
#2387=DIRECTION('center_axis',(1.,0.,-1.58362419671978E-50));
#2388=DIRECTION('ref_axis',(-1.58362419671978E-50,0.,-1.));
#2389=DIRECTION('',(-1.,0.,1.58362419671978E-50));
#2390=DIRECTION('center_axis',(1.,0.,-1.58362419671978E-50));
#2391=DIRECTION('ref_axis',(-1.58362419671978E-50,0.,-1.));
#2392=DIRECTION('center_axis',(-1.58362419671978E-50,0.,-1.));
#2393=DIRECTION('ref_axis',(-1.,0.,1.58362419671978E-50));
#2394=DIRECTION('',(-1.,0.,1.58362419671978E-50));
#2395=DIRECTION('',(0.,-1.,0.));
#2396=DIRECTION('',(0.,-1.,0.));
#2397=DIRECTION('center_axis',(-1.,0.,1.58362419671978E-50));
#2398=DIRECTION('ref_axis',(1.58362419671978E-50,0.,1.));
#2399=DIRECTION('',(-1.,0.,1.58362419671978E-50));
#2400=DIRECTION('center_axis',(1.,0.,-1.58362419671978E-50));
#2401=DIRECTION('ref_axis',(-1.58362419671978E-50,0.,-1.));
#2402=DIRECTION('center_axis',(1.,0.,-1.58362419671978E-50));
#2403=DIRECTION('ref_axis',(-1.58362419671978E-50,0.,-1.));
#2404=DIRECTION('center_axis',(0.,-1.,0.));
#2405=DIRECTION('ref_axis',(1.58362419671978E-50,0.,-1.));
#2406=DIRECTION('',(-1.,0.,1.58362419671978E-50));
#2407=DIRECTION('',(-1.58362419671978E-50,0.,1.));
#2408=DIRECTION('',(-1.58362419671978E-50,0.,1.));
#2409=DIRECTION('center_axis',(-1.,0.,1.58362419671978E-50));
#2410=DIRECTION('ref_axis',(1.58362419671978E-50,0.,1.));
#2411=DIRECTION('',(-1.,0.,1.58362419671978E-50));
#2412=DIRECTION('center_axis',(1.,0.,-1.58362419671978E-50));
#2413=DIRECTION('ref_axis',(-1.58362419671978E-50,0.,-1.));
#2414=DIRECTION('center_axis',(1.,0.,-1.58362419671978E-50));
#2415=DIRECTION('ref_axis',(-1.58362419671978E-50,0.,-1.));
#2416=DIRECTION('center_axis',(1.58362419671978E-50,0.,1.));
#2417=DIRECTION('ref_axis',(1.,0.,-1.58362419671978E-50));
#2418=DIRECTION('',(-1.,0.,1.58362419671978E-50));
#2419=DIRECTION('',(0.,1.,0.));
#2420=DIRECTION('',(0.,1.,0.));
#2421=DIRECTION('center_axis',(-1.,0.,1.58362419671978E-50));
#2422=DIRECTION('ref_axis',(1.58362419671978E-50,0.,1.));
#2423=DIRECTION('',(-1.,0.,1.58362419671978E-50));
#2424=DIRECTION('center_axis',(1.,0.,-1.58362419671978E-50));
#2425=DIRECTION('ref_axis',(-1.58362419671978E-50,0.,-1.));
#2426=DIRECTION('center_axis',(1.,0.,-1.58362419671978E-50));
#2427=DIRECTION('ref_axis',(-1.58362419671978E-50,0.,-1.));
#2428=DIRECTION('center_axis',(0.,1.,0.));
#2429=DIRECTION('ref_axis',(-1.58362419671978E-50,0.,1.));
#2430=DIRECTION('',(1.58362419671978E-50,0.,-1.));
#2431=DIRECTION('',(1.58362419671978E-50,0.,-1.));
#2432=DIRECTION('center_axis',(0.,-1.,0.));
#2433=DIRECTION('ref_axis',(1.58362419671978E-50,0.,-1.));
#2434=DIRECTION('',(-1.58362419671978E-50,0.,1.));
#2435=DIRECTION('',(-1.58362419671978E-50,0.,1.));
#2436=DIRECTION('center_axis',(1.,0.,1.58362419671978E-50));
#2437=DIRECTION('ref_axis',(1.58362419671978E-50,0.,-1.));
#2438=DIRECTION('center_axis',(1.,0.,1.58362419671978E-50));
#2439=DIRECTION('ref_axis',(1.58362419671978E-50,0.,-1.));
#2440=DIRECTION('center_axis',(1.,0.,0.));
#2441=DIRECTION('ref_axis',(0.,0.,-1.));
#2442=DIRECTION('center_axis',(1.,0.,0.));
#2443=DIRECTION('ref_axis',(0.,0.,-1.));
#2444=DIRECTION('',(0.,1.,0.));
#2445=DIRECTION('center_axis',(1.,0.,0.));
#2446=DIRECTION('ref_axis',(0.,0.,-1.));
#2447=DIRECTION('',(0.,0.,1.));
#2448=DIRECTION('center_axis',(1.,0.,0.));
#2449=DIRECTION('ref_axis',(0.,0.,-1.));
#2450=DIRECTION('',(0.,-1.,0.));
#2451=DIRECTION('center_axis',(1.,0.,0.));
#2452=DIRECTION('ref_axis',(0.,0.,-1.));
#2453=DIRECTION('',(0.,0.,-1.));
#2454=DIRECTION('center_axis',(1.,0.,0.));
#2455=DIRECTION('ref_axis',(0.,0.,-1.));
#2456=DIRECTION('',(0.,-1.,0.));
#2457=DIRECTION('center_axis',(1.,0.,0.));
#2458=DIRECTION('ref_axis',(0.,0.,-1.));
#2459=DIRECTION('',(0.,0.,-1.));
#2460=DIRECTION('center_axis',(1.,0.,0.));
#2461=DIRECTION('ref_axis',(0.,0.,-1.));
#2462=DIRECTION('',(0.,1.,0.));
#2463=DIRECTION('center_axis',(1.,0.,0.));
#2464=DIRECTION('ref_axis',(0.,0.,-1.));
#2465=DIRECTION('',(0.,0.,1.));
#2466=DIRECTION('center_axis',(1.,0.,0.));
#2467=DIRECTION('ref_axis',(0.,0.,-1.));
#2580=CARTESIAN_POINT('',(0.,0.,0.));
#2581=CARTESIAN_POINT('Origin',(280.,950.,30.));
#2582=CARTESIAN_POINT('',(280.,910.,30.));
#2583=CARTESIAN_POINT('',(280.,40.,30.));
#2584=CARTESIAN_POINT('',(280.,950.,30.));
#2585=CARTESIAN_POINT('',(280.,40.,-30.));
#2586=CARTESIAN_POINT('',(280.,40.,30.));
#2587=CARTESIAN_POINT('',(280.,910.,-30.));
#2588=CARTESIAN_POINT('',(280.,950.,-30.));
#2589=CARTESIAN_POINT('',(280.,910.,30.));
#2590=CARTESIAN_POINT('Origin',(285.,950.,30.));
#2591=CARTESIAN_POINT('',(285.,910.,35.));
#2592=CARTESIAN_POINT('',(285.,40.,35.));
#2593=CARTESIAN_POINT('',(285.,950.,35.));
#2594=CARTESIAN_POINT('Origin',(285.,40.,30.));
#2595=CARTESIAN_POINT('Origin',(285.,910.,30.));
#2596=CARTESIAN_POINT('Origin',(285.,950.,35.));
#2597=CARTESIAN_POINT('',(345.,910.,35.));
#2598=CARTESIAN_POINT('',(345.,40.,35.));
#2599=CARTESIAN_POINT('',(345.,950.,35.));
#2600=CARTESIAN_POINT('',(285.,40.,35.));
#2601=CARTESIAN_POINT('',(285.,910.,35.));
#2602=CARTESIAN_POINT('Origin',(345.,950.,30.));
#2603=CARTESIAN_POINT('',(350.,910.,30.));
#2604=CARTESIAN_POINT('',(350.,40.,30.));
#2605=CARTESIAN_POINT('',(350.,950.,30.));
#2606=CARTESIAN_POINT('Origin',(345.,40.,30.));
#2607=CARTESIAN_POINT('Origin',(345.,910.,30.));
#2608=CARTESIAN_POINT('Origin',(350.,950.,-30.));
#2609=CARTESIAN_POINT('',(350.,910.,-30.));
#2610=CARTESIAN_POINT('',(350.,40.,-30.));
#2611=CARTESIAN_POINT('',(350.,950.,-30.));
#2612=CARTESIAN_POINT('',(350.,40.,-30.));
#2613=CARTESIAN_POINT('',(350.,910.,-30.));
#2614=CARTESIAN_POINT('Origin',(345.,950.,-30.));
#2615=CARTESIAN_POINT('',(345.,910.,-35.));
#2616=CARTESIAN_POINT('',(345.,40.,-35.));
#2617=CARTESIAN_POINT('',(345.,950.,-35.));
#2618=CARTESIAN_POINT('Origin',(345.,40.,-30.));
#2619=CARTESIAN_POINT('Origin',(345.,910.,-30.));
#2620=CARTESIAN_POINT('Origin',(345.,950.,-35.));
#2621=CARTESIAN_POINT('',(285.,910.,-35.));
#2622=CARTESIAN_POINT('',(285.,40.0000000000003,-35.));
#2623=CARTESIAN_POINT('',(285.,950.,-35.));
#2624=CARTESIAN_POINT('',(345.,40.,-35.));
#2625=CARTESIAN_POINT('',(345.,910.,-35.));
#2626=CARTESIAN_POINT('Origin',(285.,950.,-30.));
#2627=CARTESIAN_POINT('Origin',(285.,40.,-30.));
#2628=CARTESIAN_POINT('Origin',(285.,910.,-30.));
#2629=CARTESIAN_POINT('Origin',(355.,950.,-30.));
#2630=CARTESIAN_POINT('',(355.,40.,-30.));
#2631=CARTESIAN_POINT('',(355.,40.,30.));
#2632=CARTESIAN_POINT('',(355.,40.,-30.));
#2633=CARTESIAN_POINT('',(355.,910.,-30.));
#2634=CARTESIAN_POINT('',(355.,950.,-30.));
#2635=CARTESIAN_POINT('',(355.,910.,30.));
#2636=CARTESIAN_POINT('',(355.,910.,-30.));
#2637=CARTESIAN_POINT('',(355.,950.,30.));
#2638=CARTESIAN_POINT('Origin',(345.,950.,30.));
#2639=CARTESIAN_POINT('',(345.,40.,40.));
#2640=CARTESIAN_POINT('Origin',(345.,40.,30.));
#2641=CARTESIAN_POINT('',(345.,910.,40.));
#2642=CARTESIAN_POINT('Origin',(345.,910.,30.));
#2643=CARTESIAN_POINT('',(345.,950.,40.));
#2644=CARTESIAN_POINT('Origin',(285.,950.,40.));
#2645=CARTESIAN_POINT('',(285.,40.,40.));
#2646=CARTESIAN_POINT('',(315.,40.,40.));
#2647=CARTESIAN_POINT('',(285.,910.,40.));
#2648=CARTESIAN_POINT('',(315.,910.,40.));
#2649=CARTESIAN_POINT('',(285.,950.,40.));
#2650=CARTESIAN_POINT('Origin',(285.,950.,30.));
#2651=CARTESIAN_POINT('',(275.,40.,30.));
#2652=CARTESIAN_POINT('Origin',(285.,40.,30.));
#2653=CARTESIAN_POINT('',(275.,910.,30.));
#2654=CARTESIAN_POINT('Origin',(285.,910.,30.));
#2655=CARTESIAN_POINT('',(275.,950.,30.));
#2656=CARTESIAN_POINT('Origin',(275.,950.,30.));
#2657=CARTESIAN_POINT('',(275.,40.,-30.));
#2658=CARTESIAN_POINT('',(275.,40.,30.));
#2659=CARTESIAN_POINT('',(275.,910.,-30.));
#2660=CARTESIAN_POINT('',(275.,910.,30.));
#2661=CARTESIAN_POINT('',(275.,950.,-30.));
#2662=CARTESIAN_POINT('Origin',(285.,950.,-30.));
#2663=CARTESIAN_POINT('',(285.,40.,-40.));
#2664=CARTESIAN_POINT('Origin',(285.,40.,-30.));
#2665=CARTESIAN_POINT('',(285.,910.,-40.));
#2666=CARTESIAN_POINT('Origin',(285.,910.,-30.));
#2667=CARTESIAN_POINT('',(285.,950.,-40.));
#2668=CARTESIAN_POINT('Origin',(345.,950.,-40.));
#2669=CARTESIAN_POINT('',(345.,40.0000000000003,-40.));
#2670=CARTESIAN_POINT('',(315.,40.,-40.));
#2671=CARTESIAN_POINT('',(345.,910.,-40.));
#2672=CARTESIAN_POINT('',(315.,910.,-40.));
#2673=CARTESIAN_POINT('',(345.,950.,-40.));
#2674=CARTESIAN_POINT('Origin',(345.,950.,-30.));
#2675=CARTESIAN_POINT('Origin',(345.,40.,-30.));
#2676=CARTESIAN_POINT('Origin',(345.,910.,-30.));
#2677=CARTESIAN_POINT('Origin',(315.,910.,-30.));
#2678=CARTESIAN_POINT('Origin',(315.,40.,30.));
#2679=CARTESIAN_POINT('Origin',(440.,950.,30.));
#2680=CARTESIAN_POINT('',(440.,910.,30.));
#2681=CARTESIAN_POINT('',(440.,40.,30.));
#2682=CARTESIAN_POINT('',(440.,950.,30.));
#2683=CARTESIAN_POINT('',(440.,40.,-30.));
#2684=CARTESIAN_POINT('',(440.,40.,30.));
#2685=CARTESIAN_POINT('',(440.,910.,-30.));
#2686=CARTESIAN_POINT('',(440.,950.,-30.));
#2687=CARTESIAN_POINT('',(440.,910.,30.));
#2688=CARTESIAN_POINT('Origin',(445.,950.,30.));
#2689=CARTESIAN_POINT('',(445.,910.,35.));
#2690=CARTESIAN_POINT('',(445.,40.,35.));
#2691=CARTESIAN_POINT('',(445.,950.,35.));
#2692=CARTESIAN_POINT('Origin',(445.,40.,30.));
#2693=CARTESIAN_POINT('Origin',(445.,910.,30.));
#2694=CARTESIAN_POINT('Origin',(445.,950.,35.));
#2695=CARTESIAN_POINT('',(505.,910.,35.));
#2696=CARTESIAN_POINT('',(505.,40.,35.));
#2697=CARTESIAN_POINT('',(505.,950.,35.));
#2698=CARTESIAN_POINT('',(445.,40.,35.));
#2699=CARTESIAN_POINT('',(445.,910.,35.));
#2700=CARTESIAN_POINT('Origin',(505.,950.,30.));
#2701=CARTESIAN_POINT('',(510.,910.,30.));
#2702=CARTESIAN_POINT('',(510.,40.,30.));
#2703=CARTESIAN_POINT('',(510.,950.,30.));
#2704=CARTESIAN_POINT('Origin',(505.,40.,30.));
#2705=CARTESIAN_POINT('Origin',(505.,910.,30.));
#2706=CARTESIAN_POINT('Origin',(510.,950.,-30.));
#2707=CARTESIAN_POINT('',(510.,910.,-30.));
#2708=CARTESIAN_POINT('',(510.,40.,-30.));
#2709=CARTESIAN_POINT('',(510.,950.,-30.));
#2710=CARTESIAN_POINT('',(510.,40.,-30.));
#2711=CARTESIAN_POINT('',(510.,910.,-30.));
#2712=CARTESIAN_POINT('Origin',(505.,950.,-30.));
#2713=CARTESIAN_POINT('',(505.,910.,-35.));
#2714=CARTESIAN_POINT('',(505.,40.,-35.));
#2715=CARTESIAN_POINT('',(505.,950.,-35.));
#2716=CARTESIAN_POINT('Origin',(505.,40.,-30.));
#2717=CARTESIAN_POINT('Origin',(505.,910.,-30.));
#2718=CARTESIAN_POINT('Origin',(505.,950.,-35.));
#2719=CARTESIAN_POINT('',(445.,910.,-35.));
#2720=CARTESIAN_POINT('',(445.,40.0000000000003,-35.));
#2721=CARTESIAN_POINT('',(445.,950.,-35.));
#2722=CARTESIAN_POINT('',(505.,40.,-35.));
#2723=CARTESIAN_POINT('',(505.,910.,-35.));
#2724=CARTESIAN_POINT('Origin',(445.,950.,-30.));
#2725=CARTESIAN_POINT('Origin',(445.,40.,-30.));
#2726=CARTESIAN_POINT('Origin',(445.,910.,-30.));
#2727=CARTESIAN_POINT('Origin',(515.,950.,-30.));
#2728=CARTESIAN_POINT('',(515.,40.,-30.));
#2729=CARTESIAN_POINT('',(515.,40.,30.));
#2730=CARTESIAN_POINT('',(515.,40.,-30.));
#2731=CARTESIAN_POINT('',(515.,910.,-30.));
#2732=CARTESIAN_POINT('',(515.,950.,-30.));
#2733=CARTESIAN_POINT('',(515.,910.,30.));
#2734=CARTESIAN_POINT('',(515.,910.,-30.));
#2735=CARTESIAN_POINT('',(515.,950.,30.));
#2736=CARTESIAN_POINT('Origin',(505.,950.,30.));
#2737=CARTESIAN_POINT('',(505.,40.,40.));
#2738=CARTESIAN_POINT('Origin',(505.,40.,30.));
#2739=CARTESIAN_POINT('',(505.,910.,40.));
#2740=CARTESIAN_POINT('Origin',(505.,910.,30.));
#2741=CARTESIAN_POINT('',(505.,950.,40.));
#2742=CARTESIAN_POINT('Origin',(445.,950.,40.));
#2743=CARTESIAN_POINT('',(445.,40.,40.));
#2744=CARTESIAN_POINT('',(475.,40.,40.));
#2745=CARTESIAN_POINT('',(445.,910.,40.));
#2746=CARTESIAN_POINT('',(475.,910.,40.));
#2747=CARTESIAN_POINT('',(445.,950.,40.));
#2748=CARTESIAN_POINT('Origin',(445.,950.,30.));
#2749=CARTESIAN_POINT('',(435.,40.,30.));
#2750=CARTESIAN_POINT('Origin',(445.,40.,30.));
#2751=CARTESIAN_POINT('',(435.,910.,30.));
#2752=CARTESIAN_POINT('Origin',(445.,910.,30.));
#2753=CARTESIAN_POINT('',(435.,950.,30.));
#2754=CARTESIAN_POINT('Origin',(435.,950.,30.));
#2755=CARTESIAN_POINT('',(435.,40.,-30.));
#2756=CARTESIAN_POINT('',(435.,40.,30.));
#2757=CARTESIAN_POINT('',(435.,910.,-30.));
#2758=CARTESIAN_POINT('',(435.,910.,30.));
#2759=CARTESIAN_POINT('',(435.,950.,-30.));
#2760=CARTESIAN_POINT('Origin',(445.,950.,-30.));
#2761=CARTESIAN_POINT('',(445.,40.,-40.));
#2762=CARTESIAN_POINT('Origin',(445.,40.,-30.));
#2763=CARTESIAN_POINT('',(445.,910.,-40.));
#2764=CARTESIAN_POINT('Origin',(445.,910.,-30.));
#2765=CARTESIAN_POINT('',(445.,950.,-40.));
#2766=CARTESIAN_POINT('Origin',(505.,950.,-40.));
#2767=CARTESIAN_POINT('',(505.,40.0000000000003,-40.));
#2768=CARTESIAN_POINT('',(475.,40.,-40.));
#2769=CARTESIAN_POINT('',(505.,910.,-40.));
#2770=CARTESIAN_POINT('',(475.,910.,-40.));
#2771=CARTESIAN_POINT('',(505.,950.,-40.));
#2772=CARTESIAN_POINT('Origin',(505.,950.,-30.));
#2773=CARTESIAN_POINT('Origin',(505.,40.,-30.));
#2774=CARTESIAN_POINT('Origin',(505.,910.,-30.));
#2775=CARTESIAN_POINT('Origin',(475.,910.,-30.));
#2776=CARTESIAN_POINT('Origin',(475.,40.,30.));
#2777=CARTESIAN_POINT('Origin',(475.,980.,30.));
#2778=CARTESIAN_POINT('',(515.,990.,30.));
#2779=CARTESIAN_POINT('',(515.,980.,40.));
#2780=CARTESIAN_POINT('Origin',(515.,980.,30.));
#2781=CARTESIAN_POINT('',(-475.,990.,30.));
#2782=CARTESIAN_POINT('',(475.,990.,30.));
#2783=CARTESIAN_POINT('',(-475.,980.,40.));
#2784=CARTESIAN_POINT('Origin',(-475.,980.,30.));
#2785=CARTESIAN_POINT('',(475.,980.,40.));
#2786=CARTESIAN_POINT('Origin',(475.,980.,40.));
#2787=CARTESIAN_POINT('',(515.,920.,40.));
#2788=CARTESIAN_POINT('',(515.,980.,40.));
#2789=CARTESIAN_POINT('',(-475.,920.,40.));
#2790=CARTESIAN_POINT('',(-475.,980.,40.));
#2791=CARTESIAN_POINT('',(475.,920.,40.));
#2792=CARTESIAN_POINT('Origin',(475.,920.,30.));
#2793=CARTESIAN_POINT('',(515.,910.,30.));
#2794=CARTESIAN_POINT('Origin',(515.,920.,30.));
#2795=CARTESIAN_POINT('',(-475.,910.,30.));
#2796=CARTESIAN_POINT('Origin',(-475.,920.,30.));
#2797=CARTESIAN_POINT('',(475.,910.,30.));
#2798=CARTESIAN_POINT('Origin',(475.,910.,-30.));
#2799=CARTESIAN_POINT('',(515.,910.,-30.));
#2800=CARTESIAN_POINT('',(515.,910.,-30.));
#2801=CARTESIAN_POINT('',(-475.,910.,-30.));
#2802=CARTESIAN_POINT('',(-475.,910.,-30.));
#2803=CARTESIAN_POINT('',(475.,910.,-30.));
#2804=CARTESIAN_POINT('Origin',(475.,920.,-30.));
#2805=CARTESIAN_POINT('',(515.,920.,-40.));
#2806=CARTESIAN_POINT('Origin',(515.,920.,-30.));
#2807=CARTESIAN_POINT('',(-475.,920.,-40.));
#2808=CARTESIAN_POINT('Origin',(-475.,920.,-30.));
#2809=CARTESIAN_POINT('',(475.,920.,-40.));
#2810=CARTESIAN_POINT('Origin',(475.,920.,-40.));
#2811=CARTESIAN_POINT('',(515.,980.,-40.));
#2812=CARTESIAN_POINT('',(515.,920.,-40.));
#2813=CARTESIAN_POINT('',(-475.,980.,-40.));
#2814=CARTESIAN_POINT('',(-475.,920.,-40.));
#2815=CARTESIAN_POINT('',(475.,980.,-40.));
#2816=CARTESIAN_POINT('Origin',(475.,980.,-30.));
#2817=CARTESIAN_POINT('',(515.,990.,-30.));
#2818=CARTESIAN_POINT('Origin',(515.,980.,-30.));
#2819=CARTESIAN_POINT('',(-475.,990.,-30.));
#2820=CARTESIAN_POINT('Origin',(-475.,980.,-30.));
#2821=CARTESIAN_POINT('',(475.,990.,-30.));
#2822=CARTESIAN_POINT('Origin',(475.,920.,30.));
#2823=CARTESIAN_POINT('',(515.,920.,35.));
#2824=CARTESIAN_POINT('',(-475.,920.,35.));
#2825=CARTESIAN_POINT('',(475.,920.,35.));
#2826=CARTESIAN_POINT('',(515.,915.,30.));
#2827=CARTESIAN_POINT('Origin',(515.,920.,30.));
#2828=CARTESIAN_POINT('',(-475.,915.,30.));
#2829=CARTESIAN_POINT('',(475.,915.,30.));
#2830=CARTESIAN_POINT('Origin',(-475.,920.,30.));
#2831=CARTESIAN_POINT('Origin',(475.,980.,35.));
#2832=CARTESIAN_POINT('',(515.,980.,35.));
#2833=CARTESIAN_POINT('',(-475.,980.,35.));
#2834=CARTESIAN_POINT('',(475.,980.,35.));
#2835=CARTESIAN_POINT('',(515.,980.,35.));
#2836=CARTESIAN_POINT('',(-475.,980.,35.));
#2837=CARTESIAN_POINT('Origin',(475.,980.,30.));
#2838=CARTESIAN_POINT('',(515.,985.,30.));
#2839=CARTESIAN_POINT('',(-475.,985.,30.));
#2840=CARTESIAN_POINT('',(475.,985.,30.));
#2841=CARTESIAN_POINT('Origin',(515.,980.,30.));
#2842=CARTESIAN_POINT('Origin',(-475.,980.,30.));
#2843=CARTESIAN_POINT('Origin',(475.,985.,30.));
#2844=CARTESIAN_POINT('',(515.,985.,-30.));
#2845=CARTESIAN_POINT('',(-475.,985.,-30.));
#2846=CARTESIAN_POINT('',(475.,985.,-30.));
#2847=CARTESIAN_POINT('',(515.,985.,30.));
#2848=CARTESIAN_POINT('',(-475.,985.,30.));
#2849=CARTESIAN_POINT('Origin',(475.,980.,-30.));
#2850=CARTESIAN_POINT('',(515.,980.,-35.));
#2851=CARTESIAN_POINT('',(-475.,980.,-35.));
#2852=CARTESIAN_POINT('',(475.,980.,-35.));
#2853=CARTESIAN_POINT('Origin',(515.,980.,-30.));
#2854=CARTESIAN_POINT('Origin',(-475.,980.,-30.));
#2855=CARTESIAN_POINT('Origin',(475.,920.,-35.));
#2856=CARTESIAN_POINT('',(515.,920.,-35.));
#2857=CARTESIAN_POINT('',(-475.,920.,-35.));
#2858=CARTESIAN_POINT('',(475.,920.,-35.));
#2859=CARTESIAN_POINT('',(515.,920.,-35.));
#2860=CARTESIAN_POINT('',(-475.,920.,-35.));
#2861=CARTESIAN_POINT('Origin',(475.,920.,-30.));
#2862=CARTESIAN_POINT('',(515.,915.,-30.));
#2863=CARTESIAN_POINT('',(-475.,915.,-30.));
#2864=CARTESIAN_POINT('',(475.,915.,-30.));
#2865=CARTESIAN_POINT('Origin',(515.,920.,-30.));
#2866=CARTESIAN_POINT('Origin',(-475.,920.,-30.));
#2867=CARTESIAN_POINT('Origin',(475.,915.,-30.));
#2868=CARTESIAN_POINT('',(515.,915.,-30.));
#2869=CARTESIAN_POINT('',(-475.,915.,-30.));
#2870=CARTESIAN_POINT('Origin',(475.,990.,30.));
#2871=CARTESIAN_POINT('',(515.,990.,30.));
#2872=CARTESIAN_POINT('',(-475.,990.,30.));
#2873=CARTESIAN_POINT('Origin',(-475.,980.,30.));
#2874=CARTESIAN_POINT('Origin',(515.,950.,-40.));
#2875=CARTESIAN_POINT('Origin',(475.,30.,30.));
#2876=CARTESIAN_POINT('',(515.,40.,30.));
#2877=CARTESIAN_POINT('',(515.,30.,40.));
#2878=CARTESIAN_POINT('Origin',(515.,30.,30.));
#2879=CARTESIAN_POINT('',(-475.,40.,30.));
#2880=CARTESIAN_POINT('',(475.,40.,30.));
#2881=CARTESIAN_POINT('',(-475.,30.,40.));
#2882=CARTESIAN_POINT('Origin',(-475.,30.,30.));
#2883=CARTESIAN_POINT('',(475.,30.,40.));
#2884=CARTESIAN_POINT('Origin',(475.,30.,40.));
#2885=CARTESIAN_POINT('',(515.,-30.,40.));
#2886=CARTESIAN_POINT('',(515.,30.,40.));
#2887=CARTESIAN_POINT('',(-475.,-30.,40.));
#2888=CARTESIAN_POINT('',(-475.,30.,40.));
#2889=CARTESIAN_POINT('',(475.,-30.,40.));
#2890=CARTESIAN_POINT('Origin',(475.,-30.,30.));
#2891=CARTESIAN_POINT('',(515.,-40.,30.));
#2892=CARTESIAN_POINT('Origin',(515.,-30.,30.));
#2893=CARTESIAN_POINT('',(-475.,-40.,30.));
#2894=CARTESIAN_POINT('Origin',(-475.,-30.,30.));
#2895=CARTESIAN_POINT('',(475.,-40.,30.));
#2896=CARTESIAN_POINT('Origin',(475.,-40.,-30.));
#2897=CARTESIAN_POINT('',(515.,-40.,-30.));
#2898=CARTESIAN_POINT('',(515.,-40.,-30.));
#2899=CARTESIAN_POINT('',(-475.,-40.,-30.));
#2900=CARTESIAN_POINT('',(-475.,-40.,-30.));
#2901=CARTESIAN_POINT('',(475.,-40.,-30.));
#2902=CARTESIAN_POINT('Origin',(475.,-30.,-30.));
#2903=CARTESIAN_POINT('',(515.,-30.,-40.));
#2904=CARTESIAN_POINT('Origin',(515.,-30.,-30.));
#2905=CARTESIAN_POINT('',(-475.,-30.,-40.));
#2906=CARTESIAN_POINT('Origin',(-475.,-30.,-30.));
#2907=CARTESIAN_POINT('',(475.,-30.,-40.));
#2908=CARTESIAN_POINT('Origin',(475.,-30.,-40.));
#2909=CARTESIAN_POINT('',(515.,30.,-40.));
#2910=CARTESIAN_POINT('',(515.,-30.,-40.));
#2911=CARTESIAN_POINT('',(-475.,30.,-40.));
#2912=CARTESIAN_POINT('',(-475.,-30.,-40.));
#2913=CARTESIAN_POINT('',(475.,30.,-40.));
#2914=CARTESIAN_POINT('Origin',(475.,30.,-30.));
#2915=CARTESIAN_POINT('',(515.,40.,-30.));
#2916=CARTESIAN_POINT('Origin',(515.,30.,-30.));
#2917=CARTESIAN_POINT('',(-475.,40.,-30.));
#2918=CARTESIAN_POINT('Origin',(-475.,30.,-30.));
#2919=CARTESIAN_POINT('',(475.,40.,-30.));
#2920=CARTESIAN_POINT('Origin',(475.,-30.,30.));
#2921=CARTESIAN_POINT('',(515.,-30.,35.));
#2922=CARTESIAN_POINT('',(-475.,-30.,35.));
#2923=CARTESIAN_POINT('',(475.,-30.,35.));
#2924=CARTESIAN_POINT('',(515.,-35.,30.));
#2925=CARTESIAN_POINT('Origin',(515.,-30.,30.));
#2926=CARTESIAN_POINT('',(-475.,-35.,30.));
#2927=CARTESIAN_POINT('',(475.,-35.,30.));
#2928=CARTESIAN_POINT('Origin',(-475.,-30.,30.));
#2929=CARTESIAN_POINT('Origin',(475.,30.,35.));
#2930=CARTESIAN_POINT('',(515.,30.,35.));
#2931=CARTESIAN_POINT('',(-475.,30.,35.));
#2932=CARTESIAN_POINT('',(475.,30.,35.));
#2933=CARTESIAN_POINT('',(515.,30.,35.));
#2934=CARTESIAN_POINT('',(-475.,30.,35.));
#2935=CARTESIAN_POINT('Origin',(475.,30.,30.));
#2936=CARTESIAN_POINT('',(515.,35.,30.));
#2937=CARTESIAN_POINT('',(-475.,35.,30.));
#2938=CARTESIAN_POINT('',(475.,35.,30.));
#2939=CARTESIAN_POINT('Origin',(515.,30.,30.));
#2940=CARTESIAN_POINT('Origin',(-475.,30.,30.));
#2941=CARTESIAN_POINT('Origin',(475.,35.,30.));
#2942=CARTESIAN_POINT('',(515.,35.,-30.));
#2943=CARTESIAN_POINT('',(-475.,35.,-30.));
#2944=CARTESIAN_POINT('',(475.,35.,-30.));
#2945=CARTESIAN_POINT('',(515.,35.,30.));
#2946=CARTESIAN_POINT('',(-475.,35.,30.));
#2947=CARTESIAN_POINT('Origin',(475.,30.,-30.));
#2948=CARTESIAN_POINT('',(515.,30.,-35.));
#2949=CARTESIAN_POINT('',(-475.,30.,-35.));
#2950=CARTESIAN_POINT('',(475.,30.,-35.));
#2951=CARTESIAN_POINT('Origin',(515.,30.,-30.));
#2952=CARTESIAN_POINT('Origin',(-475.,30.,-30.));
#2953=CARTESIAN_POINT('Origin',(475.,-30.,-35.));
#2954=CARTESIAN_POINT('',(515.,-30.,-35.));
#2955=CARTESIAN_POINT('',(-475.,-30.,-35.));
#2956=CARTESIAN_POINT('',(475.,-30.,-35.));
#2957=CARTESIAN_POINT('',(515.,-30.,-35.));
#2958=CARTESIAN_POINT('',(-475.,-30.,-35.));
#2959=CARTESIAN_POINT('Origin',(475.,-30.,-30.));
#2960=CARTESIAN_POINT('',(515.,-35.,-30.));
#2961=CARTESIAN_POINT('',(-475.,-35.,-30.));
#2962=CARTESIAN_POINT('',(475.,-35.,-30.));
#2963=CARTESIAN_POINT('Origin',(515.,-30.,-30.));
#2964=CARTESIAN_POINT('Origin',(-475.,-30.,-30.));
#2965=CARTESIAN_POINT('Origin',(475.,-35.,-30.));
#2966=CARTESIAN_POINT('',(515.,-35.,-30.));
#2967=CARTESIAN_POINT('',(-475.,-35.,-30.));
#2968=CARTESIAN_POINT('Origin',(475.,40.,30.));
#2969=CARTESIAN_POINT('',(515.,40.,30.));
#2970=CARTESIAN_POINT('',(-475.,40.,30.));
#2971=CARTESIAN_POINT('Origin',(-475.,30.,30.));
#2972=CARTESIAN_POINT('Origin',(515.,-4.89858719658941E-15,40.));
#2973=CARTESIAN_POINT('Origin',(515.,920.,-30.));
#2974=CARTESIAN_POINT('',(515.,915.,-30.));
#2975=CARTESIAN_POINT('',(515.,920.,-35.));
#2976=CARTESIAN_POINT('Origin',(515.,920.,-30.));
#2977=CARTESIAN_POINT('',(515.,980.,-35.));
#2978=CARTESIAN_POINT('',(515.,920.,-35.));
#2979=CARTESIAN_POINT('',(515.,985.,-30.));
#2980=CARTESIAN_POINT('Origin',(515.,980.,-30.));
#2981=CARTESIAN_POINT('',(515.,985.,30.));
#2982=CARTESIAN_POINT('',(515.,985.,30.));
#2983=CARTESIAN_POINT('',(515.,980.,35.));
#2984=CARTESIAN_POINT('Origin',(515.,980.,30.));
#2985=CARTESIAN_POINT('',(515.,920.,35.));
#2986=CARTESIAN_POINT('',(515.,980.,35.));
#2987=CARTESIAN_POINT('',(515.,915.,30.));
#2988=CARTESIAN_POINT('Origin',(515.,920.,30.));
#2989=CARTESIAN_POINT('',(515.,915.,-30.));
#2990=CARTESIAN_POINT('Origin',(515.,-30.,30.));
#2991=CARTESIAN_POINT('',(515.,30.,35.));
#2992=CARTESIAN_POINT('',(515.,-30.,35.));
#2993=CARTESIAN_POINT('',(515.,30.,35.));
#2994=CARTESIAN_POINT('',(515.,-35.,30.));
#2995=CARTESIAN_POINT('Origin',(515.,-30.,30.));
#2996=CARTESIAN_POINT('',(515.,-35.,-30.));
#2997=CARTESIAN_POINT('',(515.,-35.,-30.));
#2998=CARTESIAN_POINT('',(515.,-30.,-35.));
#2999=CARTESIAN_POINT('Origin',(515.,-30.,-30.));
#3000=CARTESIAN_POINT('',(515.,30.,-35.));
#3001=CARTESIAN_POINT('',(515.,-30.,-35.));
#3002=CARTESIAN_POINT('',(515.,35.,-30.));
#3003=CARTESIAN_POINT('Origin',(515.,30.,-30.));
#3004=CARTESIAN_POINT('',(515.,35.,30.));
#3005=CARTESIAN_POINT('',(515.,35.,30.));
#3006=CARTESIAN_POINT('Origin',(515.,30.,30.));
#3109=UNCERTAINTY_MEASURE_WITH_UNIT(LENGTH_MEASURE(0.01),#3120,
'DISTANCE_ACCURACY_VALUE',
'Maximum model space distance between geometric entities at asserted c
onnectivities');
#3113=UNCERTAINTY_MEASURE_WITH_UNIT(LENGTH_MEASURE(0.01),#3120,
'DISTANCE_ACCURACY_VALUE',
'Maximum model space distance between geometric entities at asserted c
onnectivities');
#3115=(
GEOMETRIC_REPRESENTATION_CONTEXT(3)
GLOBAL_UNCERTAINTY_ASSIGNED_CONTEXT((#3109))
GLOBAL_UNIT_ASSIGNED_CONTEXT((#3120,#3122,#3123))
REPRESENTATION_CONTEXT('','3D')
);
#3119=(
GEOMETRIC_REPRESENTATION_CONTEXT(3)
GLOBAL_UNCERTAINTY_ASSIGNED_CONTEXT((#3113))
GLOBAL_UNIT_ASSIGNED_CONTEXT((#3120,#3122,#3123))
REPRESENTATION_CONTEXT('','3D')
);
#3120=(
LENGTH_UNIT()
NAMED_UNIT(*)
SI_UNIT(.MILLI.,.METRE.)
);
#3122=(
NAMED_UNIT(*)
PLANE_ANGLE_UNIT()
SI_UNIT($,.RADIAN.)
);
#3123=(
NAMED_UNIT(*)
SI_UNIT($,.STERADIAN.)
SOLID_ANGLE_UNIT()
);
#3125=SHAPE_DEFINITION_REPRESENTATION(#3130,#3149);
#3130=PRODUCT_DEFINITION_SHAPE('',$,#3155);
#3149=SHAPE_REPRESENTATION('',(#1853,#77,#78),#3115);
#3153=PRODUCT_DEFINITION_CONTEXT('part definition',#3170,'design');
#3155=PRODUCT_DEFINITION('Square Tube','Square Tube',#3160,#3153);
#3160=PRODUCT_DEFINITION_FORMATION('',$,#3173);
#3170=APPLICATION_CONTEXT(
'Core Data for Automotive Mechanical Design Process');
#3171=PRODUCT_CONTEXT('part definition',#3170,'mechanical');
#3173=PRODUCT('Square Tube','Square Tube',$,(#3171));
#3178=PRESENTATION_STYLE_ASSIGNMENT((#3180));
#3180=SURFACE_STYLE_USAGE(.BOTH.,#3182);
#3182=SURFACE_SIDE_STYLE('',(#3184));
#3184=SURFACE_STYLE_FILL_AREA(#3186);
#3186=FILL_AREA_STYLE('Opaque(202,209,238)',(#3188));
#3188=FILL_AREA_STYLE_COLOUR('Opaque(202,209,238)',#3190);
#3190=COLOUR_RGB('Opaque(202,209,238)',0.792156862745098,0.819607843137255,
0.933333333333333);
ENDSEC;
END-ISO-10303-21;
